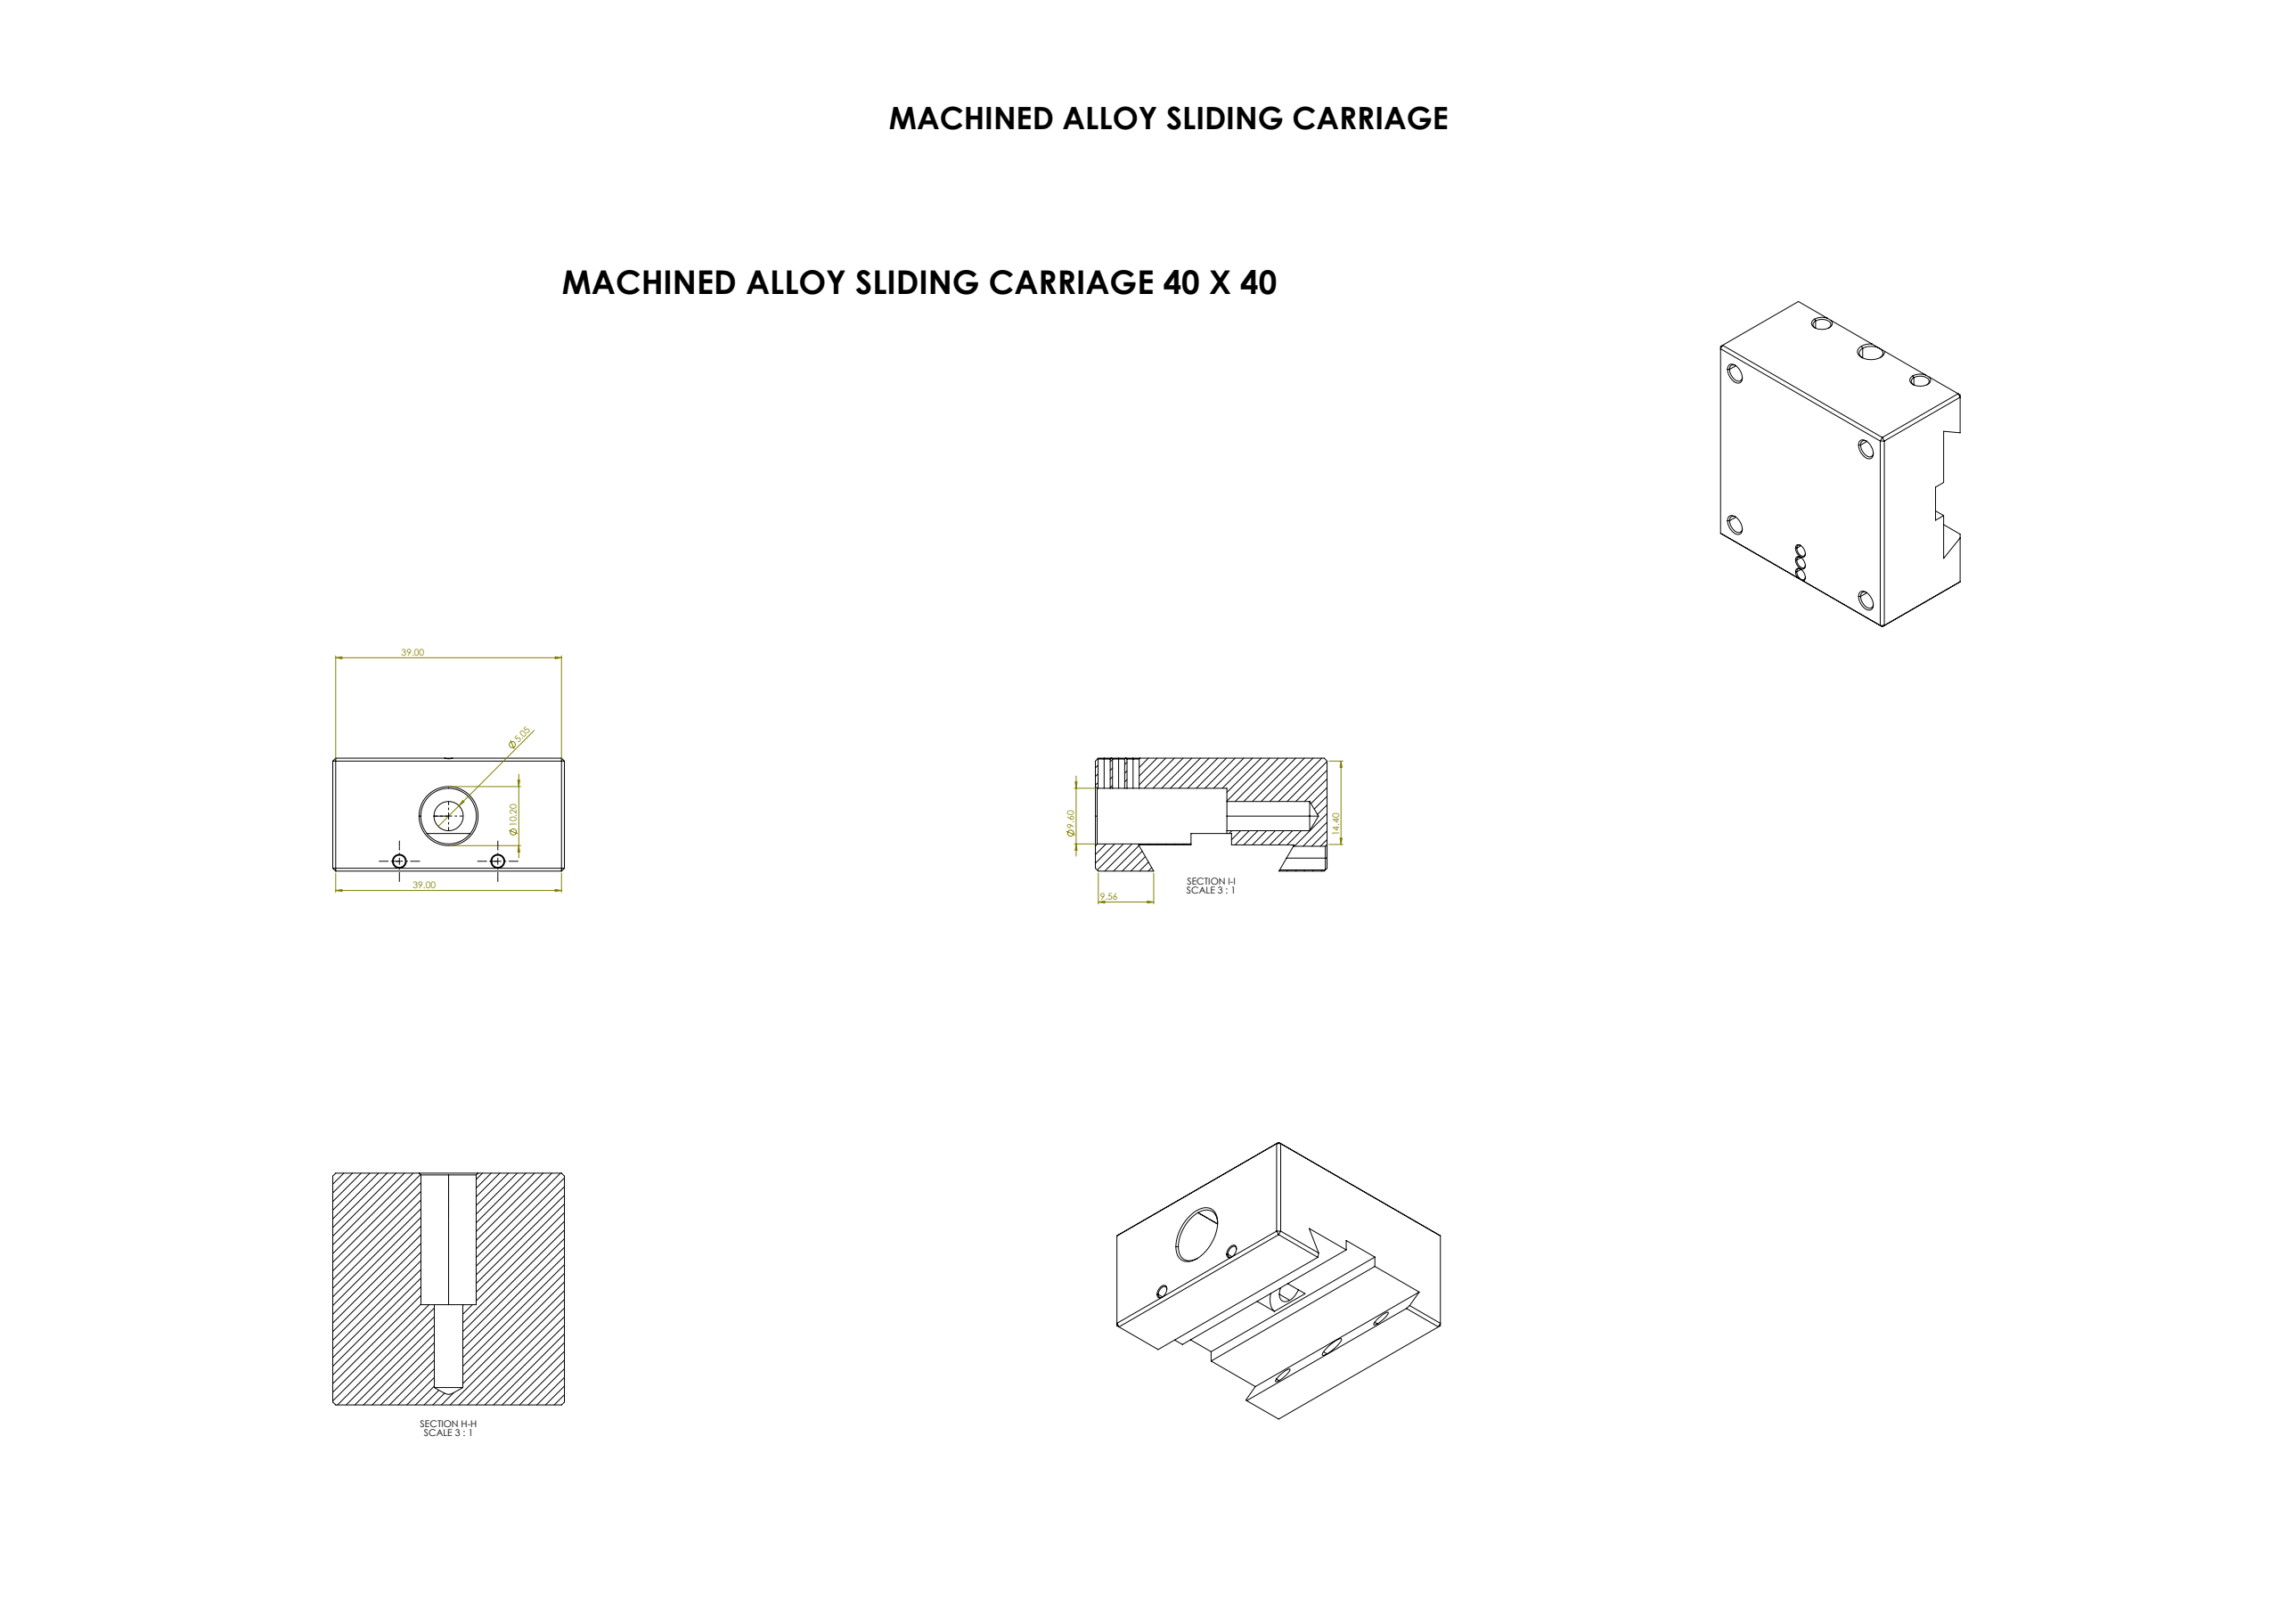
ISO-10303-21;
HEADER;
/* Generated by software containing ST-Developer
 * from STEP Tools, Inc. (www.steptools.com) 
 */

FILE_DESCRIPTION(
/* description */ (''),
/* implementation_level */ '2;1');

FILE_NAME(
/* name */ 'Machined Alloy Sliding Carriage 40 x 40.step',
/* time_stamp */ '2026-10-05T09:57:53+05:00',
/* author */ (''),
/* organization */ (''),
/* preprocessor_version */ 'ST-DEVELOPER v20.2',
/* originating_system */ 'Autodesk Translation Framework v15.15.0.0',
/* authorisation */ '');

FILE_SCHEMA (('AUTOMOTIVE_DESIGN { 1 0 10303 214 3 1 1 }'));
ENDSEC;

DATA;
#10=MECHANICAL_DESIGN_GEOMETRIC_PRESENTATION_REPRESENTATION('',(#552),#113984);
#142=(
BOUNDED_CURVE()
B_SPLINE_CURVE(2,(#92151,#92152,#92153),.UNSPECIFIED.,.F.,.F.)
B_SPLINE_CURVE_WITH_KNOTS((3,3),(0.,0.16248076809272),.UNSPECIFIED.)
CURVE()
GEOMETRIC_REPRESENTATION_ITEM()
RATIONAL_B_SPLINE_CURVE((1.,1.,1.))
REPRESENTATION_ITEM('')
);
#143=(
BOUNDED_CURVE()
B_SPLINE_CURVE(2,(#92201,#92202,#92203),.UNSPECIFIED.,.F.,.F.)
B_SPLINE_CURVE_WITH_KNOTS((3,3),(0.,0.0845576726264383),.UNSPECIFIED.)
CURVE()
GEOMETRIC_REPRESENTATION_ITEM()
RATIONAL_B_SPLINE_CURVE((1.,1.,1.))
REPRESENTATION_ITEM('')
);
#144=(
BOUNDED_CURVE()
B_SPLINE_CURVE(2,(#92222,#92223,#92224),.UNSPECIFIED.,.F.,.F.)
B_SPLINE_CURVE_WITH_KNOTS((3,3),(0.,0.0845576726264383),.UNSPECIFIED.)
CURVE()
GEOMETRIC_REPRESENTATION_ITEM()
RATIONAL_B_SPLINE_CURVE((1.,1.,1.))
REPRESENTATION_ITEM('')
);
#145=(
BOUNDED_CURVE()
B_SPLINE_CURVE(2,(#92227,#92228,#92229),.UNSPECIFIED.,.F.,.F.)
B_SPLINE_CURVE_WITH_KNOTS((3,3),(0.16248076809272,0.324961536185439),
 .UNSPECIFIED.)
CURVE()
GEOMETRIC_REPRESENTATION_ITEM()
RATIONAL_B_SPLINE_CURVE((1.,1.,1.))
REPRESENTATION_ITEM('')
);
#146=(
BOUNDED_CURVE()
B_SPLINE_CURVE(2,(#92262,#92263,#92264),.UNSPECIFIED.,.F.,.F.)
B_SPLINE_CURVE_WITH_KNOTS((3,3),(0.,0.13564659966251),.UNSPECIFIED.)
CURVE()
GEOMETRIC_REPRESENTATION_ITEM()
RATIONAL_B_SPLINE_CURVE((1.,1.,1.))
REPRESENTATION_ITEM('')
);
#516=SHAPE_REPRESENTATION_RELATIONSHIP('SRR','None',#114053,#534);
#534=ADVANCED_BREP_SHAPE_REPRESENTATION('',(#570),#113967);
#552=STYLED_ITEM('',(#114324),#570);
#570=MANIFOLD_SOLID_BREP('Machined Alloy Sliding Carriage 40 x 40',#60393);
#595=ELLIPSE('',#61838,1.78978583448783,1.54999999999999);
#596=ELLIPSE('',#61844,1.78978583448783,1.54999999999999);
#597=ELLIPSE('',#61849,2.36713610367747,2.05);
#621=CYLINDRICAL_SURFACE('',#61824,1.05);
#622=CYLINDRICAL_SURFACE('',#61828,1.05);
#623=CYLINDRICAL_SURFACE('',#61837,1.54999999999999);
#624=CYLINDRICAL_SURFACE('',#61843,1.54999999999999);
#625=CYLINDRICAL_SURFACE('',#61848,2.05);
#626=CYLINDRICAL_SURFACE('',#61856,1.05);
#627=CYLINDRICAL_SURFACE('',#61869,1.05);
#628=CYLINDRICAL_SURFACE('',#61875,1.05);
#629=CYLINDRICAL_SURFACE('',#61887,1.54999999999999);
#630=CYLINDRICAL_SURFACE('',#61891,1.54999999999999);
#631=CYLINDRICAL_SURFACE('',#61895,1.54999999999999);
#632=CYLINDRICAL_SURFACE('',#61899,1.54999999999999);
#633=CYLINDRICAL_SURFACE('',#61908,4.8);
#634=CYLINDRICAL_SURFACE('',#61914,2.525);
#887=CONICAL_SURFACE('',#61813,2.2,0.785398163397448);
#888=CONICAL_SURFACE('',#61816,1.12500000000001,0.785398163397478);
#889=CONICAL_SURFACE('',#61826,1.12500000000001,0.785398163397478);
#890=CONICAL_SURFACE('',#61830,0.525000000000002,1.02974425867666);
#891=CONICAL_SURFACE('',#61831,0.525000000000002,1.02974425867665);
#892=CONICAL_SURFACE('',#61832,1.675,0.785398163397455);
#893=CONICAL_SURFACE('',#61839,1.675,0.785398163397455);
#894=CONICAL_SURFACE('',#61845,2.2,0.785398163397448);
#895=CONICAL_SURFACE('',#61851,1.125,0.785398163397434);
#896=CONICAL_SURFACE('',#61860,1.12500000000001,0.785398163397463);
#897=CONICAL_SURFACE('',#61873,1.12500000000001,0.785398163397463);
#898=CONICAL_SURFACE('',#61885,1.675,0.785398163397457);
#899=CONICAL_SURFACE('',#61889,1.675,0.785398163397457);
#900=CONICAL_SURFACE('',#61893,1.675,0.785398163397457);
#901=CONICAL_SURFACE('',#61897,1.675,0.785398163397457);
#902=CONICAL_SURFACE('',#61901,1.54999999999999,1.02974425867665);
#903=CONICAL_SURFACE('',#61902,1.54999999999999,1.02974425867665);
#904=CONICAL_SURFACE('',#61903,1.54999999999999,1.02974425867665);
#905=CONICAL_SURFACE('',#61904,1.54999999999999,1.02974425867665);
#906=CONICAL_SURFACE('',#61905,4.95,0.785398163397434);
#907=CONICAL_SURFACE('',#61912,1.26250000000001,1.02974425867666);
#1001=CIRCLE('',#61814,2.35);
#1002=CIRCLE('',#61815,2.05);
#1003=CIRCLE('',#61817,1.20000000000001);
#1004=CIRCLE('',#61818,1.05);
#1005=CIRCLE('',#61819,1.20000000000001);
#1006=CIRCLE('',#61821,1.20000000000001);
#1007=CIRCLE('',#61822,1.20000000000001);
#1008=CIRCLE('',#61823,5.1);
#1009=CIRCLE('',#61825,1.05);
#1010=CIRCLE('',#61827,1.05);
#1011=CIRCLE('',#61829,1.05);
#1012=CIRCLE('',#61833,1.8);
#1013=CIRCLE('',#61834,1.54999999999999);
#1014=CIRCLE('',#61835,1.8);
#1015=CIRCLE('',#61840,1.8);
#1016=CIRCLE('',#61841,1.54999999999999);
#1017=CIRCLE('',#61842,1.8);
#1018=CIRCLE('',#61846,2.05);
#1019=CIRCLE('',#61847,2.35);
#1020=CIRCLE('',#61852,1.2);
#1021=CIRCLE('',#61853,1.05);
#1022=CIRCLE('',#61854,1.2);
#1023=CIRCLE('',#61857,1.05);
#1024=CIRCLE('',#61858,1.05);
#1025=CIRCLE('',#61859,1.05);
#1026=CIRCLE('',#61861,1.20000000000001);
#1027=CIRCLE('',#61862,1.05);
#1028=CIRCLE('',#61864,1.20000000000001);
#1029=CIRCLE('',#61865,1.8);
#1030=CIRCLE('',#61866,1.8);
#1031=CIRCLE('',#61867,1.8);
#1032=CIRCLE('',#61868,1.8);
#1033=CIRCLE('',#61870,1.05);
#1034=CIRCLE('',#61871,1.05);
#1035=CIRCLE('',#61872,1.05);
#1036=CIRCLE('',#61874,1.05);
#1037=CIRCLE('',#61876,1.05);
#1038=CIRCLE('',#61877,1.05);
#1039=CIRCLE('',#61878,1.05);
#1040=CIRCLE('',#61886,1.54999999999999);
#1041=CIRCLE('',#61888,1.54999999999999);
#1042=CIRCLE('',#61890,1.54999999999999);
#1043=CIRCLE('',#61892,1.54999999999999);
#1044=CIRCLE('',#61894,1.54999999999999);
#1045=CIRCLE('',#61896,1.54999999999999);
#1046=CIRCLE('',#61898,1.54999999999999);
#1047=CIRCLE('',#61900,1.54999999999999);
#1048=CIRCLE('',#61906,4.8);
#1049=CIRCLE('',#61907,4.8);
#1050=CIRCLE('',#61909,4.8);
#1051=CIRCLE('',#61910,4.8);
#1052=CIRCLE('',#61911,4.8);
#1053=CIRCLE('',#61913,2.525);
#1054=CIRCLE('',#61915,2.525);
#1811=FACE_BOUND('',#9411,.T.);
#1812=FACE_BOUND('',#9430,.T.);
#1813=FACE_BOUND('',#9431,.T.);
#1814=FACE_BOUND('',#9432,.T.);
#1815=FACE_BOUND('',#9433,.T.);
#1816=FACE_BOUND('',#9434,.T.);
#1817=FACE_BOUND('',#9435,.T.);
#1818=FACE_BOUND('',#9462,.T.);
#1819=FACE_BOUND('',#9470,.T.);
#1820=FACE_BOUND('',#9471,.T.);
#1821=FACE_BOUND('',#9472,.T.);
#2978=PLANE('',#61820);
#2979=PLANE('',#61836);
#2980=PLANE('',#61850);
#2981=PLANE('',#61855);
#2982=PLANE('',#61863);
#2983=PLANE('',#61879);
#2984=PLANE('',#61880);
#2985=PLANE('',#61881);
#2986=PLANE('',#61882);
#2987=PLANE('',#61883);
#2988=PLANE('',#61884);
#2989=PLANE('',#61916);
#2990=PLANE('',#61917);
#2991=PLANE('',#61918);
#2992=PLANE('',#61919);
#2993=PLANE('',#61920);
#2994=PLANE('',#61921);
#2995=PLANE('',#61922);
#2996=PLANE('',#61923);
#2997=PLANE('',#61924);
#2998=PLANE('',#61925);
#2999=PLANE('',#61926);
#3000=PLANE('',#61927);
#3001=PLANE('',#61928);
#3002=PLANE('',#61929);
#3003=PLANE('',#61930);
#3004=PLANE('',#61931);
#3005=PLANE('',#61932);
#3006=PLANE('',#61933);
#3007=PLANE('',#61934);
#3008=PLANE('',#61935);
#3009=PLANE('',#61936);
#3010=PLANE('',#61937);
#3011=PLANE('',#61938);
#3012=PLANE('',#61939);
#3013=PLANE('',#61940);
#3014=PLANE('',#61941);
#3015=PLANE('',#61942);
#3016=PLANE('',#61943);
#3017=PLANE('',#61944);
#3018=PLANE('',#61945);
#3019=PLANE('',#61946);
#3020=PLANE('',#61947);
#5872=FACE_OUTER_BOUND('',#9408,.T.);
#5873=FACE_OUTER_BOUND('',#9409,.T.);
#5874=FACE_OUTER_BOUND('',#9410,.T.);
#5875=FACE_OUTER_BOUND('',#9412,.T.);
#5876=FACE_OUTER_BOUND('',#9413,.T.);
#5877=FACE_OUTER_BOUND('',#9414,.T.);
#5878=FACE_OUTER_BOUND('',#9415,.T.);
#5879=FACE_OUTER_BOUND('',#9416,.T.);
#5880=FACE_OUTER_BOUND('',#9417,.T.);
#5881=FACE_OUTER_BOUND('',#9418,.T.);
#5882=FACE_OUTER_BOUND('',#9419,.T.);
#5883=FACE_OUTER_BOUND('',#9420,.T.);
#5884=FACE_OUTER_BOUND('',#9421,.T.);
#5885=FACE_OUTER_BOUND('',#9422,.T.);
#5886=FACE_OUTER_BOUND('',#9423,.T.);
#5887=FACE_OUTER_BOUND('',#9424,.T.);
#5888=FACE_OUTER_BOUND('',#9425,.T.);
#5889=FACE_OUTER_BOUND('',#9426,.T.);
#5890=FACE_OUTER_BOUND('',#9427,.T.);
#5891=FACE_OUTER_BOUND('',#9428,.T.);
#5892=FACE_OUTER_BOUND('',#9429,.T.);
#5893=FACE_OUTER_BOUND('',#9436,.T.);
#5894=FACE_OUTER_BOUND('',#9437,.T.);
#5895=FACE_OUTER_BOUND('',#9438,.T.);
#5896=FACE_OUTER_BOUND('',#9439,.T.);
#5897=FACE_OUTER_BOUND('',#9440,.T.);
#5898=FACE_OUTER_BOUND('',#9441,.T.);
#5899=FACE_OUTER_BOUND('',#9442,.T.);
#5900=FACE_OUTER_BOUND('',#9443,.T.);
#5901=FACE_OUTER_BOUND('',#9444,.T.);
#5902=FACE_OUTER_BOUND('',#9445,.T.);
#5903=FACE_OUTER_BOUND('',#9446,.T.);
#5904=FACE_OUTER_BOUND('',#9447,.T.);
#5905=FACE_OUTER_BOUND('',#9448,.T.);
#5906=FACE_OUTER_BOUND('',#9449,.T.);
#5907=FACE_OUTER_BOUND('',#9450,.T.);
#5908=FACE_OUTER_BOUND('',#9451,.T.);
#5909=FACE_OUTER_BOUND('',#9452,.T.);
#5910=FACE_OUTER_BOUND('',#9453,.T.);
#5911=FACE_OUTER_BOUND('',#9454,.T.);
#5912=FACE_OUTER_BOUND('',#9455,.T.);
#5913=FACE_OUTER_BOUND('',#9456,.T.);
#5914=FACE_OUTER_BOUND('',#9457,.T.);
#5915=FACE_OUTER_BOUND('',#9458,.T.);
#5916=FACE_OUTER_BOUND('',#9459,.T.);
#5917=FACE_OUTER_BOUND('',#9460,.T.);
#5918=FACE_OUTER_BOUND('',#9461,.T.);
#5919=FACE_OUTER_BOUND('',#9463,.T.);
#5920=FACE_OUTER_BOUND('',#9464,.T.);
#5921=FACE_OUTER_BOUND('',#9465,.T.);
#5922=FACE_OUTER_BOUND('',#9466,.T.);
#5923=FACE_OUTER_BOUND('',#9467,.T.);
#5924=FACE_OUTER_BOUND('',#9468,.T.);
#5925=FACE_OUTER_BOUND('',#9469,.T.);
#5926=FACE_OUTER_BOUND('',#9473,.T.);
#5927=FACE_OUTER_BOUND('',#9474,.T.);
#5928=FACE_OUTER_BOUND('',#9475,.T.);
#5929=FACE_OUTER_BOUND('',#9476,.T.);
#5930=FACE_OUTER_BOUND('',#9477,.T.);
#5931=FACE_OUTER_BOUND('',#9478,.T.);
#5932=FACE_OUTER_BOUND('',#9479,.T.);
#5933=FACE_OUTER_BOUND('',#9480,.T.);
#5934=FACE_OUTER_BOUND('',#9481,.T.);
#5935=FACE_OUTER_BOUND('',#9482,.T.);
#5936=FACE_OUTER_BOUND('',#9483,.T.);
#5937=FACE_OUTER_BOUND('',#9484,.T.);
#5938=FACE_OUTER_BOUND('',#9485,.T.);
#5939=FACE_OUTER_BOUND('',#9486,.T.);
#5940=FACE_OUTER_BOUND('',#9487,.T.);
#5941=FACE_OUTER_BOUND('',#9488,.T.);
#5942=FACE_OUTER_BOUND('',#9489,.T.);
#5943=FACE_OUTER_BOUND('',#9490,.T.);
#5944=FACE_OUTER_BOUND('',#9491,.T.);
#5945=FACE_OUTER_BOUND('',#9492,.T.);
#5946=FACE_OUTER_BOUND('',#9493,.T.);
#5947=FACE_OUTER_BOUND('',#9494,.T.);
#5948=FACE_OUTER_BOUND('',#9495,.T.);
#5949=FACE_OUTER_BOUND('',#9496,.T.);
#9408=EDGE_LOOP('',(#48495,#48496,#48497,#48498));
#9409=EDGE_LOOP('',(#48499,#48500,#48501,#48502,#48503));
#9410=EDGE_LOOP('',(#48504,#48505,#48506,#48507,#48508,#48509,#48510,#48511,
#48512,#48513));
#9411=EDGE_LOOP('',(#48514));
#9412=EDGE_LOOP('',(#48515,#48516,#48517,#48518));
#9413=EDGE_LOOP('',(#48519,#48520,#48521,#48522,#48523));
#9414=EDGE_LOOP('',(#48524,#48525,#48526,#48527));
#9415=EDGE_LOOP('',(#48528,#48529,#48530));
#9416=EDGE_LOOP('',(#48531,#48532,#48533));
#9417=EDGE_LOOP('',(#48534,#48535,#48536,#48537,#48538,#48539));
#9418=EDGE_LOOP('',(#48540,#48541,#48542,#48543,#48544,#48545,#48546,#48547,
#48548,#48549,#48550));
#9419=EDGE_LOOP('',(#48551,#48552,#48553,#48554));
#9420=EDGE_LOOP('',(#48555,#48556,#48557,#48558,#48559,#48560));
#9421=EDGE_LOOP('',(#48561,#48562,#48563,#48564));
#9422=EDGE_LOOP('',(#48565,#48566,#48567,#48568));
#9423=EDGE_LOOP('',(#48569,#48570,#48571,#48572,#48573));
#9424=EDGE_LOOP('',(#48574,#48575,#48576,#48577,#48578,#48579,#48580,#48581,
#48582,#48583,#48584,#48585,#48586));
#9425=EDGE_LOOP('',(#48587,#48588,#48589,#48590,#48591,#48592));
#9426=EDGE_LOOP('',(#48593,#48594,#48595,#48596,#48597,#48598));
#9427=EDGE_LOOP('',(#48599,#48600,#48601,#48602,#48603,#48604));
#9428=EDGE_LOOP('',(#48605,#48606,#48607,#48608));
#9429=EDGE_LOOP('',(#48609,#48610,#48611,#48612,#48613,#48614,#48615));
#9430=EDGE_LOOP('',(#48616));
#9431=EDGE_LOOP('',(#48617));
#9432=EDGE_LOOP('',(#48618));
#9433=EDGE_LOOP('',(#48619));
#9434=EDGE_LOOP('',(#48620));
#9435=EDGE_LOOP('',(#48621));
#9436=EDGE_LOOP('',(#48622,#48623,#48624,#48625,#48626,#48627));
#9437=EDGE_LOOP('',(#48628,#48629,#48630,#48631));
#9438=EDGE_LOOP('',(#48632,#48633,#48634,#48635,#48636,#48637));
#9439=EDGE_LOOP('',(#48638,#48639));
#9440=EDGE_LOOP('',(#48640,#48641,#48642));
#9441=EDGE_LOOP('',(#48643,#48644));
#9442=EDGE_LOOP('',(#48645,#48646,#48647));
#9443=EDGE_LOOP('',(#48648,#48649));
#9444=EDGE_LOOP('',(#48650,#48651,#48652));
#9445=EDGE_LOOP('',(#48653,#48654,#48655,#48656));
#9446=EDGE_LOOP('',(#48657,#48658,#48659,#48660));
#9447=EDGE_LOOP('',(#48661,#48662,#48663,#48664));
#9448=EDGE_LOOP('',(#48665,#48666,#48667,#48668));
#9449=EDGE_LOOP('',(#48669,#48670,#48671,#48672));
#9450=EDGE_LOOP('',(#48673,#48674,#48675,#48676));
#9451=EDGE_LOOP('',(#48677,#48678,#48679,#48680));
#9452=EDGE_LOOP('',(#48681,#48682,#48683,#48684));
#9453=EDGE_LOOP('',(#48685,#48686,#48687));
#9454=EDGE_LOOP('',(#48688,#48689,#48690));
#9455=EDGE_LOOP('',(#48691,#48692,#48693));
#9456=EDGE_LOOP('',(#48694,#48695,#48696));
#9457=EDGE_LOOP('',(#48697,#48698,#48699,#48700,#48701));
#9458=EDGE_LOOP('',(#48702,#48703,#48704,#48705,#48706,#48707,#48708,#48709,
#48710,#48711,#48712,#48713,#48714,#48715,#48716,#48717,#48718,#48719,#48720,
#48721,#48722));
#9459=EDGE_LOOP('',(#48723,#48724,#48725));
#9460=EDGE_LOOP('',(#48726,#48727,#48728,#48729));
#9461=EDGE_LOOP('',(#48730,#48731,#48732));
#9462=EDGE_LOOP('',(#48733));
#9463=EDGE_LOOP('',(#48734,#48735,#48736,#48737,#48738,#48739,#48740,#48741));
#9464=EDGE_LOOP('',(#48742,#48743,#48744,#48745));
#9465=EDGE_LOOP('',(#48746,#48747,#48748,#48749,#48750,#48751));
#9466=EDGE_LOOP('',(#48752,#48753,#48754,#48755,#48756,#48757,#48758,#48759,
#48760,#48761,#48762,#48763));
#9467=EDGE_LOOP('',(#48764,#48765,#48766,#48767));
#9468=EDGE_LOOP('',(#48768,#48769,#48770,#48771,#48772,#48773));
#9469=EDGE_LOOP('',(#48774,#48775,#48776,#48777,#48778,#48779));
#9470=EDGE_LOOP('',(#48780));
#9471=EDGE_LOOP('',(#48781));
#9472=EDGE_LOOP('',(#48782));
#9473=EDGE_LOOP('',(#48783,#48784,#48785,#48786));
#9474=EDGE_LOOP('',(#48787,#48788,#48789,#48790));
#9475=EDGE_LOOP('',(#48791,#48792,#48793,#48794));
#9476=EDGE_LOOP('',(#48795,#48796,#48797,#48798));
#9477=EDGE_LOOP('',(#48799,#48800,#48801,#48802));
#9478=EDGE_LOOP('',(#48803,#48804,#48805));
#9479=EDGE_LOOP('',(#48806,#48807,#48808));
#9480=EDGE_LOOP('',(#48809,#48810,#48811));
#9481=EDGE_LOOP('',(#48812,#48813,#48814));
#9482=EDGE_LOOP('',(#48815,#48816,#48817));
#9483=EDGE_LOOP('',(#48818,#48819,#48820));
#9484=EDGE_LOOP('',(#48821,#48822,#48823));
#9485=EDGE_LOOP('',(#48824,#48825,#48826));
#9486=EDGE_LOOP('',(#48827,#48828,#48829,#48830));
#9487=EDGE_LOOP('',(#48831,#48832,#48833,#48834));
#9488=EDGE_LOOP('',(#48835,#48836,#48837,#48838));
#9489=EDGE_LOOP('',(#48839,#48840,#48841,#48842));
#9490=EDGE_LOOP('',(#48843,#48844,#48845,#48846));
#9491=EDGE_LOOP('',(#48847,#48848,#48849,#48850));
#9492=EDGE_LOOP('',(#48851,#48852,#48853,#48854));
#9493=EDGE_LOOP('',(#48855,#48856,#48857,#48858,#48859,#48860));
#9494=EDGE_LOOP('',(#48861,#48862,#48863,#48864));
#9495=EDGE_LOOP('',(#48865,#48866,#48867,#48868));
#9496=EDGE_LOOP('',(#48869,#48870,#48871,#48872,#48873,#48874,#48875,#48876,
#48877,#48878,#48879,#48880));
#14156=LINE('',#92147,#20190);
#14157=LINE('',#92160,#20191);
#14158=LINE('',#92166,#20192);
#14159=LINE('',#92168,#20193);
#14160=LINE('',#92172,#20194);
#14161=LINE('',#92174,#20195);
#14162=LINE('',#92176,#20196);
#14163=LINE('',#92177,#20197);
#14164=LINE('',#92182,#20198);
#14165=LINE('',#92186,#20199);
#14166=LINE('',#92190,#20200);
#14167=LINE('',#92194,#20201);
#14168=LINE('',#92197,#20202);
#14169=LINE('',#92207,#20203);
#14170=LINE('',#92212,#20204);
#14171=LINE('',#92214,#20205);
#14172=LINE('',#92216,#20206);
#14173=LINE('',#92218,#20207);
#14174=LINE('',#92220,#20208);
#14175=LINE('',#92226,#20209);
#14176=LINE('',#92230,#20210);
#14177=LINE('',#92233,#20211);
#14178=LINE('',#92239,#20212);
#14179=LINE('',#92244,#20213);
#14180=LINE('',#92251,#20214);
#14181=LINE('',#92255,#20215);
#14182=LINE('',#92257,#20216);
#14183=LINE('',#92258,#20217);
#14184=LINE('',#92268,#20218);
#14185=LINE('',#92273,#20219);
#14186=LINE('',#92274,#20220);
#14187=LINE('',#92276,#20221);
#14188=LINE('',#92277,#20222);
#14189=LINE('',#92280,#20223);
#14190=LINE('',#92290,#20224);
#14191=LINE('',#92294,#20225);
#14192=LINE('',#92296,#20226);
#14193=LINE('',#92297,#20227);
#14194=LINE('',#92310,#20228);
#14195=LINE('',#92318,#20229);
#14196=LINE('',#92322,#20230);
#14197=LINE('',#92329,#20231);
#14198=LINE('',#92331,#20232);
#14199=LINE('',#92333,#20233);
#14200=LINE('',#92335,#20234);
#14201=LINE('',#92337,#20235);
#14202=LINE('',#92339,#20236);
#14203=LINE('',#92342,#20237);
#14204=LINE('',#92346,#20238);
#14205=LINE('',#92350,#20239);
#14206=LINE('',#92354,#20240);
#14207=LINE('',#92358,#20241);
#14208=LINE('',#92362,#20242);
#14209=LINE('',#92366,#20243);
#14210=LINE('',#92370,#20244);
#14211=LINE('',#92374,#20245);
#14212=LINE('',#92377,#20246);
#14213=LINE('',#92380,#20247);
#14214=LINE('',#92383,#20248);
#14215=LINE('',#92386,#20249);
#14216=LINE('',#92391,#20250);
#14217=LINE('',#92392,#20251);
#14218=LINE('',#92393,#20252);
#14219=LINE('',#92395,#20253);
#14220=LINE('',#92399,#20254);
#14221=LINE('',#92403,#20255);
#14222=LINE('',#92408,#20256);
#14223=LINE('',#92413,#20257);
#14224=LINE('',#92415,#20258);
#14225=LINE('',#92418,#20259);
#14226=LINE('',#92420,#20260);
#14227=LINE('',#92422,#20261);
#14228=LINE('',#92424,#20262);
#14229=LINE('',#92425,#20263);
#14230=LINE('',#92429,#20264);
#14231=LINE('',#92430,#20265);
#14232=LINE('',#92431,#20266);
#14233=LINE('',#92434,#20267);
#14234=LINE('',#92436,#20268);
#14235=LINE('',#92437,#20269);
#14236=LINE('',#92440,#20270);
#14237=LINE('',#92442,#20271);
#14238=LINE('',#92444,#20272);
#14239=LINE('',#92446,#20273);
#14240=LINE('',#92448,#20274);
#14241=LINE('',#92450,#20275);
#14242=LINE('',#92452,#20276);
#14243=LINE('',#92454,#20277);
#14244=LINE('',#92455,#20278);
#14245=LINE('',#92458,#20279);
#14246=LINE('',#92459,#20280);
#14247=LINE('',#92462,#20281);
#14248=LINE('',#92464,#20282);
#14249=LINE('',#92466,#20283);
#14250=LINE('',#92467,#20284);
#14251=LINE('',#92470,#20285);
#14252=LINE('',#92472,#20286);
#14253=LINE('',#92474,#20287);
#14254=LINE('',#92476,#20288);
#14255=LINE('',#92477,#20289);
#14256=LINE('',#92479,#20290);
#14257=LINE('',#92482,#20291);
#14258=LINE('',#92483,#20292);
#14259=LINE('',#92485,#20293);
#14260=LINE('',#92486,#20294);
#14261=LINE('',#92489,#20295);
#14262=LINE('',#92490,#20296);
#14263=LINE('',#92493,#20297);
#14264=LINE('',#92494,#20298);
#14265=LINE('',#92496,#20299);
#14266=LINE('',#92497,#20300);
#14267=LINE('',#92500,#20301);
#14268=LINE('',#92501,#20302);
#14269=LINE('',#92503,#20303);
#14270=LINE('',#92504,#20304);
#14271=LINE('',#92507,#20305);
#14272=LINE('',#92508,#20306);
#14273=LINE('',#92510,#20307);
#14274=LINE('',#92511,#20308);
#14275=LINE('',#92514,#20309);
#14276=LINE('',#92515,#20310);
#14277=LINE('',#92516,#20311);
#14278=LINE('',#92518,#20312);
#14279=LINE('',#92520,#20313);
#14280=LINE('',#92521,#20314);
#14281=LINE('',#92522,#20315);
#14282=LINE('',#92527,#20316);
#14283=LINE('',#92529,#20317);
#14284=LINE('',#92532,#20318);
#14285=LINE('',#92533,#20319);
#14286=LINE('',#92536,#20320);
#20190=VECTOR('',#69466,2.2);
#20191=VECTOR('',#69475,1.12500000000001);
#20192=VECTOR('',#69482,10.);
#20193=VECTOR('',#69483,10.);
#20194=VECTOR('',#69488,10.);
#20195=VECTOR('',#69489,10.);
#20196=VECTOR('',#69490,10.);
#20197=VECTOR('',#69491,10.);
#20198=VECTOR('',#69496,1.05);
#20199=VECTOR('',#69501,1.12500000000001);
#20200=VECTOR('',#69506,1.05);
#20201=VECTOR('',#69511,0.525000000000002);
#20202=VECTOR('',#69514,0.525000000000002);
#20203=VECTOR('',#69519,1.675);
#20204=VECTOR('',#69526,10.);
#20205=VECTOR('',#69527,10.);
#20206=VECTOR('',#69528,10.);
#20207=VECTOR('',#69529,10.);
#20208=VECTOR('',#69530,10.);
#20209=VECTOR('',#69531,10.);
#20210=VECTOR('',#69532,10.);
#20211=VECTOR('',#69535,1.54999999999999);
#20212=VECTOR('',#69542,1.675);
#20213=VECTOR('',#69549,1.54999999999999);
#20214=VECTOR('',#69560,2.05);
#20215=VECTOR('',#69565,10.);
#20216=VECTOR('',#69566,10.);
#20217=VECTOR('',#69567,10.);
#20218=VECTOR('',#69572,1.125);
#20219=VECTOR('',#69579,10.);
#20220=VECTOR('',#69580,10.);
#20221=VECTOR('',#69581,10.);
#20222=VECTOR('',#69582,10.);
#20223=VECTOR('',#69585,1.05);
#20224=VECTOR('',#69596,1.12500000000001);
#20225=VECTOR('',#69601,10.);
#20226=VECTOR('',#69602,10.);
#20227=VECTOR('',#69603,10.);
#20228=VECTOR('',#69616,1.05);
#20229=VECTOR('',#69625,1.12500000000001);
#20230=VECTOR('',#69630,1.05);
#20231=VECTOR('',#69639,10.);
#20232=VECTOR('',#69642,10.);
#20233=VECTOR('',#69645,10.);
#20234=VECTOR('',#69648,10.);
#20235=VECTOR('',#69651,10.);
#20236=VECTOR('',#69654,10.);
#20237=VECTOR('',#69657,1.675);
#20238=VECTOR('',#69662,1.54999999999999);
#20239=VECTOR('',#69667,1.675);
#20240=VECTOR('',#69672,1.54999999999999);
#20241=VECTOR('',#69677,1.675);
#20242=VECTOR('',#69682,1.54999999999999);
#20243=VECTOR('',#69687,1.675);
#20244=VECTOR('',#69692,1.54999999999999);
#20245=VECTOR('',#69697,1.54999999999999);
#20246=VECTOR('',#69700,1.54999999999999);
#20247=VECTOR('',#69703,1.54999999999999);
#20248=VECTOR('',#69706,1.54999999999999);
#20249=VECTOR('',#69709,4.95);
#20250=VECTOR('',#69716,4.8);
#20251=VECTOR('',#69717,4.8);
#20252=VECTOR('',#69718,4.8);
#20253=VECTOR('',#69719,4.8);
#20254=VECTOR('',#69722,10.);
#20255=VECTOR('',#69725,10.);
#20256=VECTOR('',#69730,1.26250000000001);
#20257=VECTOR('',#69737,2.525);
#20258=VECTOR('',#69740,10.);
#20259=VECTOR('',#69743,10.);
#20260=VECTOR('',#69744,10.);
#20261=VECTOR('',#69745,10.);
#20262=VECTOR('',#69746,10.);
#20263=VECTOR('',#69747,10.);
#20264=VECTOR('',#69750,10.);
#20265=VECTOR('',#69751,10.);
#20266=VECTOR('',#69752,10.);
#20267=VECTOR('',#69755,10.);
#20268=VECTOR('',#69756,10.);
#20269=VECTOR('',#69757,10.);
#20270=VECTOR('',#69760,10.);
#20271=VECTOR('',#69761,10.);
#20272=VECTOR('',#69762,10.);
#20273=VECTOR('',#69763,10.);
#20274=VECTOR('',#69764,10.);
#20275=VECTOR('',#69765,10.);
#20276=VECTOR('',#69766,10.);
#20277=VECTOR('',#69767,10.);
#20278=VECTOR('',#69768,10.);
#20279=VECTOR('',#69771,10.);
#20280=VECTOR('',#69772,10.);
#20281=VECTOR('',#69775,10.);
#20282=VECTOR('',#69776,10.);
#20283=VECTOR('',#69777,10.);
#20284=VECTOR('',#69778,10.);
#20285=VECTOR('',#69781,10.);
#20286=VECTOR('',#69782,10.);
#20287=VECTOR('',#69783,10.);
#20288=VECTOR('',#69784,10.);
#20289=VECTOR('',#69785,10.);
#20290=VECTOR('',#69788,10.);
#20291=VECTOR('',#69791,10.);
#20292=VECTOR('',#69792,10.);
#20293=VECTOR('',#69795,10.);
#20294=VECTOR('',#69796,10.);
#20295=VECTOR('',#69799,10.);
#20296=VECTOR('',#69800,10.);
#20297=VECTOR('',#69803,10.);
#20298=VECTOR('',#69804,10.);
#20299=VECTOR('',#69807,10.);
#20300=VECTOR('',#69808,10.);
#20301=VECTOR('',#69811,10.);
#20302=VECTOR('',#69812,10.);
#20303=VECTOR('',#69815,10.);
#20304=VECTOR('',#69816,10.);
#20305=VECTOR('',#69819,10.);
#20306=VECTOR('',#69820,10.);
#20307=VECTOR('',#69823,10.);
#20308=VECTOR('',#69824,10.);
#20309=VECTOR('',#69827,10.);
#20310=VECTOR('',#69828,10.);
#20311=VECTOR('',#69829,10.);
#20312=VECTOR('',#69832,10.);
#20313=VECTOR('',#69835,10.);
#20314=VECTOR('',#69836,10.);
#20315=VECTOR('',#69837,10.);
#20316=VECTOR('',#69846,10.);
#20317=VECTOR('',#69849,10.);
#20318=VECTOR('',#69854,10.);
#20319=VECTOR('',#69855,10.);
#20320=VECTOR('',#69860,10.);
#27763=VERTEX_POINT('',#92145);
#27764=VERTEX_POINT('',#92146);
#27765=VERTEX_POINT('',#92148);
#27766=VERTEX_POINT('',#92150);
#27767=VERTEX_POINT('',#92156);
#27768=VERTEX_POINT('',#92157);
#27769=VERTEX_POINT('',#92159);
#27770=VERTEX_POINT('',#92164);
#27771=VERTEX_POINT('',#92165);
#27772=VERTEX_POINT('',#92167);
#27773=VERTEX_POINT('',#92169);
#27774=VERTEX_POINT('',#92173);
#27775=VERTEX_POINT('',#92175);
#27776=VERTEX_POINT('',#92178);
#27777=VERTEX_POINT('',#92181);
#27778=VERTEX_POINT('',#92185);
#27779=VERTEX_POINT('',#92189);
#27780=VERTEX_POINT('',#92193);
#27781=VERTEX_POINT('',#92196);
#27782=VERTEX_POINT('',#92199);
#27783=VERTEX_POINT('',#92200);
#27784=VERTEX_POINT('',#92204);
#27785=VERTEX_POINT('',#92206);
#27786=VERTEX_POINT('',#92211);
#27787=VERTEX_POINT('',#92213);
#27788=VERTEX_POINT('',#92215);
#27789=VERTEX_POINT('',#92217);
#27790=VERTEX_POINT('',#92219);
#27791=VERTEX_POINT('',#92221);
#27792=VERTEX_POINT('',#92225);
#27793=VERTEX_POINT('',#92232);
#27794=VERTEX_POINT('',#92236);
#27795=VERTEX_POINT('',#92238);
#27796=VERTEX_POINT('',#92243);
#27797=VERTEX_POINT('',#92250);
#27798=VERTEX_POINT('',#92254);
#27799=VERTEX_POINT('',#92256);
#27800=VERTEX_POINT('',#92260);
#27801=VERTEX_POINT('',#92261);
#27802=VERTEX_POINT('',#92265);
#27803=VERTEX_POINT('',#92267);
#27804=VERTEX_POINT('',#92272);
#27805=VERTEX_POINT('',#92275);
#27806=VERTEX_POINT('',#92279);
#27807=VERTEX_POINT('',#92281);
#27808=VERTEX_POINT('',#92283);
#27809=VERTEX_POINT('',#92287);
#27810=VERTEX_POINT('',#92289);
#27811=VERTEX_POINT('',#92293);
#27812=VERTEX_POINT('',#92295);
#27813=VERTEX_POINT('',#92298);
#27814=VERTEX_POINT('',#92300);
#27815=VERTEX_POINT('',#92302);
#27816=VERTEX_POINT('',#92304);
#27817=VERTEX_POINT('',#92306);
#27818=VERTEX_POINT('',#92309);
#27819=VERTEX_POINT('',#92311);
#27820=VERTEX_POINT('',#92313);
#27821=VERTEX_POINT('',#92317);
#27822=VERTEX_POINT('',#92321);
#27823=VERTEX_POINT('',#92323);
#27824=VERTEX_POINT('',#92325);
#27825=VERTEX_POINT('',#92341);
#27826=VERTEX_POINT('',#92345);
#27827=VERTEX_POINT('',#92349);
#27828=VERTEX_POINT('',#92353);
#27829=VERTEX_POINT('',#92357);
#27830=VERTEX_POINT('',#92361);
#27831=VERTEX_POINT('',#92365);
#27832=VERTEX_POINT('',#92369);
#27833=VERTEX_POINT('',#92373);
#27834=VERTEX_POINT('',#92376);
#27835=VERTEX_POINT('',#92379);
#27836=VERTEX_POINT('',#92382);
#27837=VERTEX_POINT('',#92385);
#27838=VERTEX_POINT('',#92387);
#27839=VERTEX_POINT('',#92394);
#27840=VERTEX_POINT('',#92396);
#27841=VERTEX_POINT('',#92398);
#27842=VERTEX_POINT('',#92400);
#27843=VERTEX_POINT('',#92402);
#27844=VERTEX_POINT('',#92406);
#27845=VERTEX_POINT('',#92407);
#27846=VERTEX_POINT('',#92411);
#27847=VERTEX_POINT('',#92417);
#27848=VERTEX_POINT('',#92419);
#27849=VERTEX_POINT('',#92421);
#27850=VERTEX_POINT('',#92423);
#27851=VERTEX_POINT('',#92427);
#27852=VERTEX_POINT('',#92428);
#27853=VERTEX_POINT('',#92433);
#27854=VERTEX_POINT('',#92435);
#27855=VERTEX_POINT('',#92439);
#27856=VERTEX_POINT('',#92441);
#27857=VERTEX_POINT('',#92443);
#27858=VERTEX_POINT('',#92445);
#27859=VERTEX_POINT('',#92447);
#27860=VERTEX_POINT('',#92449);
#27861=VERTEX_POINT('',#92451);
#27862=VERTEX_POINT('',#92453);
#27863=VERTEX_POINT('',#92457);
#27864=VERTEX_POINT('',#92461);
#27865=VERTEX_POINT('',#92463);
#27866=VERTEX_POINT('',#92465);
#27867=VERTEX_POINT('',#92469);
#27868=VERTEX_POINT('',#92471);
#27869=VERTEX_POINT('',#92473);
#27870=VERTEX_POINT('',#92475);
#27871=VERTEX_POINT('',#92481);
#27872=VERTEX_POINT('',#92488);
#27873=VERTEX_POINT('',#92492);
#27874=VERTEX_POINT('',#92499);
#27875=VERTEX_POINT('',#92506);
#27876=VERTEX_POINT('',#92513);
#35080=EDGE_CURVE('',#27763,#27764,#14156,.T.);
#35081=EDGE_CURVE('',#27763,#27765,#1001,.T.);
#35082=EDGE_CURVE('',#27765,#27766,#142,.T.);
#35083=EDGE_CURVE('',#27766,#27764,#1002,.T.);
#35084=EDGE_CURVE('',#27767,#27768,#1003,.T.);
#35085=EDGE_CURVE('',#27768,#27769,#14157,.T.);
#35086=EDGE_CURVE('',#27769,#27769,#1004,.T.);
#35087=EDGE_CURVE('',#27768,#27767,#1005,.T.);
#35088=EDGE_CURVE('',#27770,#27771,#14158,.T.);
#35089=EDGE_CURVE('',#27772,#27770,#14159,.T.);
#35090=EDGE_CURVE('',#27773,#27772,#1006,.T.);
#35091=EDGE_CURVE('',#27772,#27773,#1007,.T.);
#35092=EDGE_CURVE('',#27767,#27772,#14160,.T.);
#35093=EDGE_CURVE('',#27774,#27767,#14161,.T.);
#35094=EDGE_CURVE('',#27775,#27774,#14162,.T.);
#35095=EDGE_CURVE('',#27771,#27775,#14163,.T.);
#35096=EDGE_CURVE('',#27776,#27776,#1008,.T.);
#35097=EDGE_CURVE('',#27769,#27777,#14164,.T.);
#35098=EDGE_CURVE('',#27777,#27777,#1009,.T.);
#35099=EDGE_CURVE('',#27773,#27778,#14165,.T.);
#35100=EDGE_CURVE('',#27778,#27778,#1010,.T.);
#35101=EDGE_CURVE('',#27778,#27779,#14166,.T.);
#35102=EDGE_CURVE('',#27779,#27779,#1011,.T.);
#35103=EDGE_CURVE('',#27780,#27777,#14167,.T.);
#35104=EDGE_CURVE('',#27781,#27779,#14168,.T.);
#35105=EDGE_CURVE('',#27782,#27783,#143,.T.);
#35106=EDGE_CURVE('',#27783,#27784,#1012,.T.);
#35107=EDGE_CURVE('',#27784,#27785,#14169,.T.);
#35108=EDGE_CURVE('',#27785,#27785,#1013,.T.);
#35109=EDGE_CURVE('',#27784,#27782,#1014,.T.);
#35110=EDGE_CURVE('',#27782,#27786,#14170,.T.);
#35111=EDGE_CURVE('',#27786,#27787,#14171,.T.);
#35112=EDGE_CURVE('',#27787,#27788,#14172,.T.);
#35113=EDGE_CURVE('',#27788,#27789,#14173,.T.);
#35114=EDGE_CURVE('',#27789,#27790,#14174,.T.);
#35115=EDGE_CURVE('',#27791,#27790,#144,.T.);
#35116=EDGE_CURVE('',#27791,#27792,#14175,.T.);
#35117=EDGE_CURVE('',#27766,#27792,#145,.T.);
#35118=EDGE_CURVE('',#27765,#27783,#14176,.T.);
#35119=EDGE_CURVE('',#27785,#27793,#14177,.T.);
#35120=EDGE_CURVE('',#27793,#27793,#595,.T.);
#35121=EDGE_CURVE('',#27790,#27794,#1015,.T.);
#35122=EDGE_CURVE('',#27794,#27795,#14178,.T.);
#35123=EDGE_CURVE('',#27795,#27795,#1016,.T.);
#35124=EDGE_CURVE('',#27794,#27791,#1017,.T.);
#35125=EDGE_CURVE('',#27795,#27796,#14179,.T.);
#35126=EDGE_CURVE('',#27796,#27796,#596,.T.);
#35127=EDGE_CURVE('',#27764,#27766,#1018,.T.);
#35128=EDGE_CURVE('',#27792,#27763,#1019,.T.);
#35129=EDGE_CURVE('',#27764,#27797,#14180,.T.);
#35130=EDGE_CURVE('',#27797,#27797,#597,.T.);
#35131=EDGE_CURVE('',#27798,#27789,#14181,.T.);
#35132=EDGE_CURVE('',#27799,#27798,#14182,.T.);
#35133=EDGE_CURVE('',#27786,#27799,#14183,.T.);
#35134=EDGE_CURVE('',#27800,#27801,#146,.T.);
#35135=EDGE_CURVE('',#27801,#27802,#1020,.T.);
#35136=EDGE_CURVE('',#27802,#27803,#14184,.T.);
#35137=EDGE_CURVE('',#27803,#27803,#1021,.T.);
#35138=EDGE_CURVE('',#27802,#27800,#1022,.T.);
#35139=EDGE_CURVE('',#27800,#27804,#14185,.T.);
#35140=EDGE_CURVE('',#27804,#27771,#14186,.T.);
#35141=EDGE_CURVE('',#27775,#27805,#14187,.T.);
#35142=EDGE_CURVE('',#27805,#27801,#14188,.T.);
#35143=EDGE_CURVE('',#27803,#27806,#14189,.T.);
#35144=EDGE_CURVE('',#27806,#27807,#1023,.T.);
#35145=EDGE_CURVE('',#27807,#27808,#1024,.T.);
#35146=EDGE_CURVE('',#27808,#27806,#1025,.T.);
#35147=EDGE_CURVE('',#27809,#27809,#1026,.T.);
#35148=EDGE_CURVE('',#27809,#27810,#14190,.T.);
#35149=EDGE_CURVE('',#27810,#27810,#1027,.T.);
#35150=EDGE_CURVE('',#27811,#27805,#14191,.T.);
#35151=EDGE_CURVE('',#27812,#27811,#14192,.T.);
#35152=EDGE_CURVE('',#27804,#27812,#14193,.T.);
#35153=EDGE_CURVE('',#27813,#27813,#1028,.T.);
#35154=EDGE_CURVE('',#27814,#27814,#1029,.T.);
#35155=EDGE_CURVE('',#27815,#27815,#1030,.T.);
#35156=EDGE_CURVE('',#27816,#27816,#1031,.T.);
#35157=EDGE_CURVE('',#27817,#27817,#1032,.T.);
#35158=EDGE_CURVE('',#27810,#27818,#14194,.T.);
#35159=EDGE_CURVE('',#27818,#27819,#1033,.T.);
#35160=EDGE_CURVE('',#27819,#27820,#1034,.T.);
#35161=EDGE_CURVE('',#27820,#27818,#1035,.T.);
#35162=EDGE_CURVE('',#27813,#27821,#14195,.T.);
#35163=EDGE_CURVE('',#27821,#27821,#1036,.T.);
#35164=EDGE_CURVE('',#27821,#27822,#14196,.T.);
#35165=EDGE_CURVE('',#27822,#27823,#1037,.T.);
#35166=EDGE_CURVE('',#27823,#27824,#1038,.T.);
#35167=EDGE_CURVE('',#27824,#27822,#1039,.T.);
#35168=EDGE_CURVE('',#27823,#27824,#14197,.T.);
#35169=EDGE_CURVE('',#27823,#27824,#14198,.T.);
#35170=EDGE_CURVE('',#27819,#27820,#14199,.T.);
#35171=EDGE_CURVE('',#27819,#27820,#14200,.T.);
#35172=EDGE_CURVE('',#27807,#27808,#14201,.T.);
#35173=EDGE_CURVE('',#27807,#27808,#14202,.T.);
#35174=EDGE_CURVE('',#27814,#27825,#14203,.T.);
#35175=EDGE_CURVE('',#27825,#27825,#1040,.T.);
#35176=EDGE_CURVE('',#27825,#27826,#14204,.T.);
#35177=EDGE_CURVE('',#27826,#27826,#1041,.T.);
#35178=EDGE_CURVE('',#27817,#27827,#14205,.T.);
#35179=EDGE_CURVE('',#27827,#27827,#1042,.T.);
#35180=EDGE_CURVE('',#27827,#27828,#14206,.T.);
#35181=EDGE_CURVE('',#27828,#27828,#1043,.T.);
#35182=EDGE_CURVE('',#27815,#27829,#14207,.T.);
#35183=EDGE_CURVE('',#27829,#27829,#1044,.T.);
#35184=EDGE_CURVE('',#27829,#27830,#14208,.T.);
#35185=EDGE_CURVE('',#27830,#27830,#1045,.T.);
#35186=EDGE_CURVE('',#27816,#27831,#14209,.T.);
#35187=EDGE_CURVE('',#27831,#27831,#1046,.T.);
#35188=EDGE_CURVE('',#27831,#27832,#14210,.T.);
#35189=EDGE_CURVE('',#27832,#27832,#1047,.T.);
#35190=EDGE_CURVE('',#27826,#27833,#14211,.T.);
#35191=EDGE_CURVE('',#27832,#27834,#14212,.T.);
#35192=EDGE_CURVE('',#27830,#27835,#14213,.T.);
#35193=EDGE_CURVE('',#27828,#27836,#14214,.T.);
#35194=EDGE_CURVE('',#27776,#27837,#14215,.T.);
#35195=EDGE_CURVE('',#27837,#27838,#1048,.T.);
#35196=EDGE_CURVE('',#27838,#27837,#1049,.T.);
#35197=EDGE_CURVE('',#27838,#27808,#14216,.T.);
#35198=EDGE_CURVE('',#27807,#27820,#14217,.T.);
#35199=EDGE_CURVE('',#27819,#27824,#14218,.T.);
#35200=EDGE_CURVE('',#27823,#27839,#14219,.T.);
#35201=EDGE_CURVE('',#27839,#27840,#1050,.T.);
#35202=EDGE_CURVE('',#27841,#27840,#14220,.T.);
#35203=EDGE_CURVE('',#27842,#27841,#1051,.T.);
#35204=EDGE_CURVE('',#27843,#27842,#14221,.T.);
#35205=EDGE_CURVE('',#27843,#27839,#1052,.T.);
#35206=EDGE_CURVE('',#27844,#27845,#14222,.T.);
#35207=EDGE_CURVE('',#27845,#27845,#1053,.T.);
#35208=EDGE_CURVE('',#27846,#27846,#1054,.T.);
#35209=EDGE_CURVE('',#27846,#27845,#14223,.T.);
#35210=EDGE_CURVE('',#27840,#27843,#14224,.T.);
#35211=EDGE_CURVE('',#27847,#27842,#14225,.T.);
#35212=EDGE_CURVE('',#27848,#27847,#14226,.T.);
#35213=EDGE_CURVE('',#27848,#27849,#14227,.T.);
#35214=EDGE_CURVE('',#27850,#27849,#14228,.T.);
#35215=EDGE_CURVE('',#27841,#27850,#14229,.T.);
#35216=EDGE_CURVE('',#27851,#27852,#14230,.T.);
#35217=EDGE_CURVE('',#27849,#27851,#14231,.T.);
#35218=EDGE_CURVE('',#27852,#27848,#14232,.T.);
#35219=EDGE_CURVE('',#27853,#27850,#14233,.T.);
#35220=EDGE_CURVE('',#27854,#27853,#14234,.T.);
#35221=EDGE_CURVE('',#27847,#27854,#14235,.T.);
#35222=EDGE_CURVE('',#27854,#27855,#14236,.T.);
#35223=EDGE_CURVE('',#27855,#27856,#14237,.T.);
#35224=EDGE_CURVE('',#27857,#27856,#14238,.T.);
#35225=EDGE_CURVE('',#27858,#27857,#14239,.T.);
#35226=EDGE_CURVE('',#27859,#27858,#14240,.T.);
#35227=EDGE_CURVE('',#27860,#27859,#14241,.T.);
#35228=EDGE_CURVE('',#27861,#27860,#14242,.T.);
#35229=EDGE_CURVE('',#27861,#27862,#14243,.T.);
#35230=EDGE_CURVE('',#27862,#27852,#14244,.T.);
#35231=EDGE_CURVE('',#27863,#27853,#14245,.T.);
#35232=EDGE_CURVE('',#27855,#27863,#14246,.T.);
#35233=EDGE_CURVE('',#27856,#27864,#14247,.T.);
#35234=EDGE_CURVE('',#27865,#27863,#14248,.T.);
#35235=EDGE_CURVE('',#27866,#27865,#14249,.T.);
#35236=EDGE_CURVE('',#27864,#27866,#14250,.T.);
#35237=EDGE_CURVE('',#27867,#27861,#14251,.T.);
#35238=EDGE_CURVE('',#27868,#27867,#14252,.T.);
#35239=EDGE_CURVE('',#27869,#27868,#14253,.T.);
#35240=EDGE_CURVE('',#27870,#27869,#14254,.T.);
#35241=EDGE_CURVE('',#27862,#27870,#14255,.T.);
#35242=EDGE_CURVE('',#27851,#27870,#14256,.T.);
#35243=EDGE_CURVE('',#27864,#27871,#14257,.T.);
#35244=EDGE_CURVE('',#27871,#27857,#14258,.T.);
#35245=EDGE_CURVE('',#27860,#27788,#14259,.T.);
#35246=EDGE_CURVE('',#27788,#27867,#14260,.T.);
#35247=EDGE_CURVE('',#27872,#27866,#14261,.T.);
#35248=EDGE_CURVE('',#27871,#27872,#14262,.T.);
#35249=EDGE_CURVE('',#27865,#27873,#14263,.T.);
#35250=EDGE_CURVE('',#27873,#27872,#14264,.T.);
#35251=EDGE_CURVE('',#27774,#27873,#14265,.T.);
#35252=EDGE_CURVE('',#27872,#27774,#14266,.T.);
#35253=EDGE_CURVE('',#27805,#27874,#14267,.T.);
#35254=EDGE_CURVE('',#27874,#27775,#14268,.T.);
#35255=EDGE_CURVE('',#27770,#27871,#14269,.T.);
#35256=EDGE_CURVE('',#27857,#27770,#14270,.T.);
#35257=EDGE_CURVE('',#27787,#27875,#14271,.T.);
#35258=EDGE_CURVE('',#27875,#27786,#14272,.T.);
#35259=EDGE_CURVE('',#27858,#27804,#14273,.T.);
#35260=EDGE_CURVE('',#27771,#27858,#14274,.T.);
#35261=EDGE_CURVE('',#27799,#27876,#14275,.T.);
#35262=EDGE_CURVE('',#27811,#27799,#14276,.T.);
#35263=EDGE_CURVE('',#27876,#27811,#14277,.T.);
#35264=EDGE_CURVE('',#27789,#27860,#14278,.T.);
#35265=EDGE_CURVE('',#27859,#27798,#14279,.T.);
#35266=EDGE_CURVE('',#27812,#27859,#14280,.T.);
#35267=EDGE_CURVE('',#27798,#27812,#14281,.T.);
#35268=EDGE_CURVE('',#27874,#27876,#14282,.T.);
#35269=EDGE_CURVE('',#27876,#27875,#14283,.T.);
#35270=EDGE_CURVE('',#27868,#27787,#14284,.T.);
#35271=EDGE_CURVE('',#27875,#27869,#14285,.T.);
#35272=EDGE_CURVE('',#27873,#27874,#14286,.T.);
#48495=ORIENTED_EDGE('',*,*,#35080,.F.);
#48496=ORIENTED_EDGE('',*,*,#35081,.T.);
#48497=ORIENTED_EDGE('',*,*,#35082,.T.);
#48498=ORIENTED_EDGE('',*,*,#35083,.T.);
#48499=ORIENTED_EDGE('',*,*,#35084,.T.);
#48500=ORIENTED_EDGE('',*,*,#35085,.T.);
#48501=ORIENTED_EDGE('',*,*,#35086,.T.);
#48502=ORIENTED_EDGE('',*,*,#35085,.F.);
#48503=ORIENTED_EDGE('',*,*,#35087,.T.);
#48504=ORIENTED_EDGE('',*,*,#35088,.F.);
#48505=ORIENTED_EDGE('',*,*,#35089,.F.);
#48506=ORIENTED_EDGE('',*,*,#35090,.F.);
#48507=ORIENTED_EDGE('',*,*,#35091,.F.);
#48508=ORIENTED_EDGE('',*,*,#35092,.F.);
#48509=ORIENTED_EDGE('',*,*,#35087,.F.);
#48510=ORIENTED_EDGE('',*,*,#35084,.F.);
#48511=ORIENTED_EDGE('',*,*,#35093,.F.);
#48512=ORIENTED_EDGE('',*,*,#35094,.F.);
#48513=ORIENTED_EDGE('',*,*,#35095,.F.);
#48514=ORIENTED_EDGE('',*,*,#35096,.F.);
#48515=ORIENTED_EDGE('',*,*,#35086,.F.);
#48516=ORIENTED_EDGE('',*,*,#35097,.T.);
#48517=ORIENTED_EDGE('',*,*,#35098,.T.);
#48518=ORIENTED_EDGE('',*,*,#35097,.F.);
#48519=ORIENTED_EDGE('',*,*,#35091,.T.);
#48520=ORIENTED_EDGE('',*,*,#35099,.T.);
#48521=ORIENTED_EDGE('',*,*,#35100,.T.);
#48522=ORIENTED_EDGE('',*,*,#35099,.F.);
#48523=ORIENTED_EDGE('',*,*,#35090,.T.);
#48524=ORIENTED_EDGE('',*,*,#35100,.F.);
#48525=ORIENTED_EDGE('',*,*,#35101,.T.);
#48526=ORIENTED_EDGE('',*,*,#35102,.T.);
#48527=ORIENTED_EDGE('',*,*,#35101,.F.);
#48528=ORIENTED_EDGE('',*,*,#35103,.T.);
#48529=ORIENTED_EDGE('',*,*,#35098,.F.);
#48530=ORIENTED_EDGE('',*,*,#35103,.F.);
#48531=ORIENTED_EDGE('',*,*,#35104,.T.);
#48532=ORIENTED_EDGE('',*,*,#35102,.F.);
#48533=ORIENTED_EDGE('',*,*,#35104,.F.);
#48534=ORIENTED_EDGE('',*,*,#35105,.T.);
#48535=ORIENTED_EDGE('',*,*,#35106,.T.);
#48536=ORIENTED_EDGE('',*,*,#35107,.T.);
#48537=ORIENTED_EDGE('',*,*,#35108,.T.);
#48538=ORIENTED_EDGE('',*,*,#35107,.F.);
#48539=ORIENTED_EDGE('',*,*,#35109,.T.);
#48540=ORIENTED_EDGE('',*,*,#35105,.F.);
#48541=ORIENTED_EDGE('',*,*,#35110,.T.);
#48542=ORIENTED_EDGE('',*,*,#35111,.T.);
#48543=ORIENTED_EDGE('',*,*,#35112,.T.);
#48544=ORIENTED_EDGE('',*,*,#35113,.T.);
#48545=ORIENTED_EDGE('',*,*,#35114,.T.);
#48546=ORIENTED_EDGE('',*,*,#35115,.F.);
#48547=ORIENTED_EDGE('',*,*,#35116,.T.);
#48548=ORIENTED_EDGE('',*,*,#35117,.F.);
#48549=ORIENTED_EDGE('',*,*,#35082,.F.);
#48550=ORIENTED_EDGE('',*,*,#35118,.T.);
#48551=ORIENTED_EDGE('',*,*,#35108,.F.);
#48552=ORIENTED_EDGE('',*,*,#35119,.T.);
#48553=ORIENTED_EDGE('',*,*,#35120,.F.);
#48554=ORIENTED_EDGE('',*,*,#35119,.F.);
#48555=ORIENTED_EDGE('',*,*,#35115,.T.);
#48556=ORIENTED_EDGE('',*,*,#35121,.T.);
#48557=ORIENTED_EDGE('',*,*,#35122,.T.);
#48558=ORIENTED_EDGE('',*,*,#35123,.T.);
#48559=ORIENTED_EDGE('',*,*,#35122,.F.);
#48560=ORIENTED_EDGE('',*,*,#35124,.T.);
#48561=ORIENTED_EDGE('',*,*,#35123,.F.);
#48562=ORIENTED_EDGE('',*,*,#35125,.T.);
#48563=ORIENTED_EDGE('',*,*,#35126,.F.);
#48564=ORIENTED_EDGE('',*,*,#35125,.F.);
#48565=ORIENTED_EDGE('',*,*,#35080,.T.);
#48566=ORIENTED_EDGE('',*,*,#35127,.T.);
#48567=ORIENTED_EDGE('',*,*,#35117,.T.);
#48568=ORIENTED_EDGE('',*,*,#35128,.T.);
#48569=ORIENTED_EDGE('',*,*,#35083,.F.);
#48570=ORIENTED_EDGE('',*,*,#35127,.F.);
#48571=ORIENTED_EDGE('',*,*,#35129,.T.);
#48572=ORIENTED_EDGE('',*,*,#35130,.F.);
#48573=ORIENTED_EDGE('',*,*,#35129,.F.);
#48574=ORIENTED_EDGE('',*,*,#35106,.F.);
#48575=ORIENTED_EDGE('',*,*,#35118,.F.);
#48576=ORIENTED_EDGE('',*,*,#35081,.F.);
#48577=ORIENTED_EDGE('',*,*,#35128,.F.);
#48578=ORIENTED_EDGE('',*,*,#35116,.F.);
#48579=ORIENTED_EDGE('',*,*,#35124,.F.);
#48580=ORIENTED_EDGE('',*,*,#35121,.F.);
#48581=ORIENTED_EDGE('',*,*,#35114,.F.);
#48582=ORIENTED_EDGE('',*,*,#35131,.F.);
#48583=ORIENTED_EDGE('',*,*,#35132,.F.);
#48584=ORIENTED_EDGE('',*,*,#35133,.F.);
#48585=ORIENTED_EDGE('',*,*,#35110,.F.);
#48586=ORIENTED_EDGE('',*,*,#35109,.F.);
#48587=ORIENTED_EDGE('',*,*,#35134,.T.);
#48588=ORIENTED_EDGE('',*,*,#35135,.T.);
#48589=ORIENTED_EDGE('',*,*,#35136,.T.);
#48590=ORIENTED_EDGE('',*,*,#35137,.T.);
#48591=ORIENTED_EDGE('',*,*,#35136,.F.);
#48592=ORIENTED_EDGE('',*,*,#35138,.T.);
#48593=ORIENTED_EDGE('',*,*,#35134,.F.);
#48594=ORIENTED_EDGE('',*,*,#35139,.T.);
#48595=ORIENTED_EDGE('',*,*,#35140,.T.);
#48596=ORIENTED_EDGE('',*,*,#35095,.T.);
#48597=ORIENTED_EDGE('',*,*,#35141,.T.);
#48598=ORIENTED_EDGE('',*,*,#35142,.T.);
#48599=ORIENTED_EDGE('',*,*,#35137,.F.);
#48600=ORIENTED_EDGE('',*,*,#35143,.T.);
#48601=ORIENTED_EDGE('',*,*,#35144,.T.);
#48602=ORIENTED_EDGE('',*,*,#35145,.T.);
#48603=ORIENTED_EDGE('',*,*,#35146,.T.);
#48604=ORIENTED_EDGE('',*,*,#35143,.F.);
#48605=ORIENTED_EDGE('',*,*,#35147,.T.);
#48606=ORIENTED_EDGE('',*,*,#35148,.T.);
#48607=ORIENTED_EDGE('',*,*,#35149,.T.);
#48608=ORIENTED_EDGE('',*,*,#35148,.F.);
#48609=ORIENTED_EDGE('',*,*,#35135,.F.);
#48610=ORIENTED_EDGE('',*,*,#35142,.F.);
#48611=ORIENTED_EDGE('',*,*,#35150,.F.);
#48612=ORIENTED_EDGE('',*,*,#35151,.F.);
#48613=ORIENTED_EDGE('',*,*,#35152,.F.);
#48614=ORIENTED_EDGE('',*,*,#35139,.F.);
#48615=ORIENTED_EDGE('',*,*,#35138,.F.);
#48616=ORIENTED_EDGE('',*,*,#35153,.F.);
#48617=ORIENTED_EDGE('',*,*,#35154,.F.);
#48618=ORIENTED_EDGE('',*,*,#35155,.F.);
#48619=ORIENTED_EDGE('',*,*,#35156,.F.);
#48620=ORIENTED_EDGE('',*,*,#35157,.F.);
#48621=ORIENTED_EDGE('',*,*,#35147,.F.);
#48622=ORIENTED_EDGE('',*,*,#35149,.F.);
#48623=ORIENTED_EDGE('',*,*,#35158,.T.);
#48624=ORIENTED_EDGE('',*,*,#35159,.T.);
#48625=ORIENTED_EDGE('',*,*,#35160,.T.);
#48626=ORIENTED_EDGE('',*,*,#35161,.T.);
#48627=ORIENTED_EDGE('',*,*,#35158,.F.);
#48628=ORIENTED_EDGE('',*,*,#35153,.T.);
#48629=ORIENTED_EDGE('',*,*,#35162,.T.);
#48630=ORIENTED_EDGE('',*,*,#35163,.T.);
#48631=ORIENTED_EDGE('',*,*,#35162,.F.);
#48632=ORIENTED_EDGE('',*,*,#35163,.F.);
#48633=ORIENTED_EDGE('',*,*,#35164,.T.);
#48634=ORIENTED_EDGE('',*,*,#35165,.T.);
#48635=ORIENTED_EDGE('',*,*,#35166,.T.);
#48636=ORIENTED_EDGE('',*,*,#35167,.T.);
#48637=ORIENTED_EDGE('',*,*,#35164,.F.);
#48638=ORIENTED_EDGE('',*,*,#35168,.T.);
#48639=ORIENTED_EDGE('',*,*,#35166,.F.);
#48640=ORIENTED_EDGE('',*,*,#35169,.F.);
#48641=ORIENTED_EDGE('',*,*,#35165,.F.);
#48642=ORIENTED_EDGE('',*,*,#35167,.F.);
#48643=ORIENTED_EDGE('',*,*,#35170,.T.);
#48644=ORIENTED_EDGE('',*,*,#35160,.F.);
#48645=ORIENTED_EDGE('',*,*,#35171,.F.);
#48646=ORIENTED_EDGE('',*,*,#35159,.F.);
#48647=ORIENTED_EDGE('',*,*,#35161,.F.);
#48648=ORIENTED_EDGE('',*,*,#35172,.T.);
#48649=ORIENTED_EDGE('',*,*,#35145,.F.);
#48650=ORIENTED_EDGE('',*,*,#35173,.F.);
#48651=ORIENTED_EDGE('',*,*,#35144,.F.);
#48652=ORIENTED_EDGE('',*,*,#35146,.F.);
#48653=ORIENTED_EDGE('',*,*,#35154,.T.);
#48654=ORIENTED_EDGE('',*,*,#35174,.T.);
#48655=ORIENTED_EDGE('',*,*,#35175,.T.);
#48656=ORIENTED_EDGE('',*,*,#35174,.F.);
#48657=ORIENTED_EDGE('',*,*,#35175,.F.);
#48658=ORIENTED_EDGE('',*,*,#35176,.T.);
#48659=ORIENTED_EDGE('',*,*,#35177,.T.);
#48660=ORIENTED_EDGE('',*,*,#35176,.F.);
#48661=ORIENTED_EDGE('',*,*,#35157,.T.);
#48662=ORIENTED_EDGE('',*,*,#35178,.T.);
#48663=ORIENTED_EDGE('',*,*,#35179,.T.);
#48664=ORIENTED_EDGE('',*,*,#35178,.F.);
#48665=ORIENTED_EDGE('',*,*,#35179,.F.);
#48666=ORIENTED_EDGE('',*,*,#35180,.T.);
#48667=ORIENTED_EDGE('',*,*,#35181,.T.);
#48668=ORIENTED_EDGE('',*,*,#35180,.F.);
#48669=ORIENTED_EDGE('',*,*,#35155,.T.);
#48670=ORIENTED_EDGE('',*,*,#35182,.T.);
#48671=ORIENTED_EDGE('',*,*,#35183,.T.);
#48672=ORIENTED_EDGE('',*,*,#35182,.F.);
#48673=ORIENTED_EDGE('',*,*,#35183,.F.);
#48674=ORIENTED_EDGE('',*,*,#35184,.T.);
#48675=ORIENTED_EDGE('',*,*,#35185,.T.);
#48676=ORIENTED_EDGE('',*,*,#35184,.F.);
#48677=ORIENTED_EDGE('',*,*,#35156,.T.);
#48678=ORIENTED_EDGE('',*,*,#35186,.T.);
#48679=ORIENTED_EDGE('',*,*,#35187,.T.);
#48680=ORIENTED_EDGE('',*,*,#35186,.F.);
#48681=ORIENTED_EDGE('',*,*,#35187,.F.);
#48682=ORIENTED_EDGE('',*,*,#35188,.T.);
#48683=ORIENTED_EDGE('',*,*,#35189,.T.);
#48684=ORIENTED_EDGE('',*,*,#35188,.F.);
#48685=ORIENTED_EDGE('',*,*,#35177,.F.);
#48686=ORIENTED_EDGE('',*,*,#35190,.T.);
#48687=ORIENTED_EDGE('',*,*,#35190,.F.);
#48688=ORIENTED_EDGE('',*,*,#35189,.F.);
#48689=ORIENTED_EDGE('',*,*,#35191,.T.);
#48690=ORIENTED_EDGE('',*,*,#35191,.F.);
#48691=ORIENTED_EDGE('',*,*,#35185,.F.);
#48692=ORIENTED_EDGE('',*,*,#35192,.T.);
#48693=ORIENTED_EDGE('',*,*,#35192,.F.);
#48694=ORIENTED_EDGE('',*,*,#35181,.F.);
#48695=ORIENTED_EDGE('',*,*,#35193,.T.);
#48696=ORIENTED_EDGE('',*,*,#35193,.F.);
#48697=ORIENTED_EDGE('',*,*,#35096,.T.);
#48698=ORIENTED_EDGE('',*,*,#35194,.T.);
#48699=ORIENTED_EDGE('',*,*,#35195,.T.);
#48700=ORIENTED_EDGE('',*,*,#35196,.T.);
#48701=ORIENTED_EDGE('',*,*,#35194,.F.);
#48702=ORIENTED_EDGE('',*,*,#35195,.F.);
#48703=ORIENTED_EDGE('',*,*,#35196,.F.);
#48704=ORIENTED_EDGE('',*,*,#35197,.T.);
#48705=ORIENTED_EDGE('',*,*,#35172,.F.);
#48706=ORIENTED_EDGE('',*,*,#35198,.T.);
#48707=ORIENTED_EDGE('',*,*,#35170,.F.);
#48708=ORIENTED_EDGE('',*,*,#35199,.T.);
#48709=ORIENTED_EDGE('',*,*,#35168,.F.);
#48710=ORIENTED_EDGE('',*,*,#35200,.T.);
#48711=ORIENTED_EDGE('',*,*,#35201,.T.);
#48712=ORIENTED_EDGE('',*,*,#35202,.F.);
#48713=ORIENTED_EDGE('',*,*,#35203,.F.);
#48714=ORIENTED_EDGE('',*,*,#35204,.F.);
#48715=ORIENTED_EDGE('',*,*,#35205,.T.);
#48716=ORIENTED_EDGE('',*,*,#35200,.F.);
#48717=ORIENTED_EDGE('',*,*,#35169,.T.);
#48718=ORIENTED_EDGE('',*,*,#35199,.F.);
#48719=ORIENTED_EDGE('',*,*,#35171,.T.);
#48720=ORIENTED_EDGE('',*,*,#35198,.F.);
#48721=ORIENTED_EDGE('',*,*,#35173,.T.);
#48722=ORIENTED_EDGE('',*,*,#35197,.F.);
#48723=ORIENTED_EDGE('',*,*,#35206,.T.);
#48724=ORIENTED_EDGE('',*,*,#35207,.F.);
#48725=ORIENTED_EDGE('',*,*,#35206,.F.);
#48726=ORIENTED_EDGE('',*,*,#35208,.F.);
#48727=ORIENTED_EDGE('',*,*,#35209,.T.);
#48728=ORIENTED_EDGE('',*,*,#35207,.T.);
#48729=ORIENTED_EDGE('',*,*,#35209,.F.);
#48730=ORIENTED_EDGE('',*,*,#35210,.F.);
#48731=ORIENTED_EDGE('',*,*,#35201,.F.);
#48732=ORIENTED_EDGE('',*,*,#35205,.F.);
#48733=ORIENTED_EDGE('',*,*,#35208,.T.);
#48734=ORIENTED_EDGE('',*,*,#35202,.T.);
#48735=ORIENTED_EDGE('',*,*,#35210,.T.);
#48736=ORIENTED_EDGE('',*,*,#35204,.T.);
#48737=ORIENTED_EDGE('',*,*,#35211,.F.);
#48738=ORIENTED_EDGE('',*,*,#35212,.F.);
#48739=ORIENTED_EDGE('',*,*,#35213,.T.);
#48740=ORIENTED_EDGE('',*,*,#35214,.F.);
#48741=ORIENTED_EDGE('',*,*,#35215,.F.);
#48742=ORIENTED_EDGE('',*,*,#35216,.F.);
#48743=ORIENTED_EDGE('',*,*,#35217,.F.);
#48744=ORIENTED_EDGE('',*,*,#35213,.F.);
#48745=ORIENTED_EDGE('',*,*,#35218,.F.);
#48746=ORIENTED_EDGE('',*,*,#35203,.T.);
#48747=ORIENTED_EDGE('',*,*,#35215,.T.);
#48748=ORIENTED_EDGE('',*,*,#35219,.F.);
#48749=ORIENTED_EDGE('',*,*,#35220,.F.);
#48750=ORIENTED_EDGE('',*,*,#35221,.F.);
#48751=ORIENTED_EDGE('',*,*,#35211,.T.);
#48752=ORIENTED_EDGE('',*,*,#35218,.T.);
#48753=ORIENTED_EDGE('',*,*,#35212,.T.);
#48754=ORIENTED_EDGE('',*,*,#35221,.T.);
#48755=ORIENTED_EDGE('',*,*,#35222,.T.);
#48756=ORIENTED_EDGE('',*,*,#35223,.T.);
#48757=ORIENTED_EDGE('',*,*,#35224,.F.);
#48758=ORIENTED_EDGE('',*,*,#35225,.F.);
#48759=ORIENTED_EDGE('',*,*,#35226,.F.);
#48760=ORIENTED_EDGE('',*,*,#35227,.F.);
#48761=ORIENTED_EDGE('',*,*,#35228,.F.);
#48762=ORIENTED_EDGE('',*,*,#35229,.T.);
#48763=ORIENTED_EDGE('',*,*,#35230,.T.);
#48764=ORIENTED_EDGE('',*,*,#35220,.T.);
#48765=ORIENTED_EDGE('',*,*,#35231,.F.);
#48766=ORIENTED_EDGE('',*,*,#35232,.F.);
#48767=ORIENTED_EDGE('',*,*,#35222,.F.);
#48768=ORIENTED_EDGE('',*,*,#35233,.F.);
#48769=ORIENTED_EDGE('',*,*,#35223,.F.);
#48770=ORIENTED_EDGE('',*,*,#35232,.T.);
#48771=ORIENTED_EDGE('',*,*,#35234,.F.);
#48772=ORIENTED_EDGE('',*,*,#35235,.F.);
#48773=ORIENTED_EDGE('',*,*,#35236,.F.);
#48774=ORIENTED_EDGE('',*,*,#35237,.F.);
#48775=ORIENTED_EDGE('',*,*,#35238,.F.);
#48776=ORIENTED_EDGE('',*,*,#35239,.F.);
#48777=ORIENTED_EDGE('',*,*,#35240,.F.);
#48778=ORIENTED_EDGE('',*,*,#35241,.F.);
#48779=ORIENTED_EDGE('',*,*,#35229,.F.);
#48780=ORIENTED_EDGE('',*,*,#35126,.T.);
#48781=ORIENTED_EDGE('',*,*,#35120,.T.);
#48782=ORIENTED_EDGE('',*,*,#35130,.T.);
#48783=ORIENTED_EDGE('',*,*,#35216,.T.);
#48784=ORIENTED_EDGE('',*,*,#35230,.F.);
#48785=ORIENTED_EDGE('',*,*,#35241,.T.);
#48786=ORIENTED_EDGE('',*,*,#35242,.F.);
#48787=ORIENTED_EDGE('',*,*,#35233,.T.);
#48788=ORIENTED_EDGE('',*,*,#35243,.T.);
#48789=ORIENTED_EDGE('',*,*,#35244,.T.);
#48790=ORIENTED_EDGE('',*,*,#35224,.T.);
#48791=ORIENTED_EDGE('',*,*,#35237,.T.);
#48792=ORIENTED_EDGE('',*,*,#35228,.T.);
#48793=ORIENTED_EDGE('',*,*,#35245,.T.);
#48794=ORIENTED_EDGE('',*,*,#35246,.T.);
#48795=ORIENTED_EDGE('',*,*,#35236,.T.);
#48796=ORIENTED_EDGE('',*,*,#35247,.F.);
#48797=ORIENTED_EDGE('',*,*,#35248,.F.);
#48798=ORIENTED_EDGE('',*,*,#35243,.F.);
#48799=ORIENTED_EDGE('',*,*,#35235,.T.);
#48800=ORIENTED_EDGE('',*,*,#35249,.T.);
#48801=ORIENTED_EDGE('',*,*,#35250,.T.);
#48802=ORIENTED_EDGE('',*,*,#35247,.T.);
#48803=ORIENTED_EDGE('',*,*,#35251,.F.);
#48804=ORIENTED_EDGE('',*,*,#35252,.F.);
#48805=ORIENTED_EDGE('',*,*,#35250,.F.);
#48806=ORIENTED_EDGE('',*,*,#35253,.F.);
#48807=ORIENTED_EDGE('',*,*,#35141,.F.);
#48808=ORIENTED_EDGE('',*,*,#35254,.F.);
#48809=ORIENTED_EDGE('',*,*,#35255,.F.);
#48810=ORIENTED_EDGE('',*,*,#35256,.F.);
#48811=ORIENTED_EDGE('',*,*,#35244,.F.);
#48812=ORIENTED_EDGE('',*,*,#35257,.F.);
#48813=ORIENTED_EDGE('',*,*,#35111,.F.);
#48814=ORIENTED_EDGE('',*,*,#35258,.F.);
#48815=ORIENTED_EDGE('',*,*,#35140,.F.);
#48816=ORIENTED_EDGE('',*,*,#35259,.F.);
#48817=ORIENTED_EDGE('',*,*,#35260,.F.);
#48818=ORIENTED_EDGE('',*,*,#35261,.F.);
#48819=ORIENTED_EDGE('',*,*,#35262,.F.);
#48820=ORIENTED_EDGE('',*,*,#35263,.F.);
#48821=ORIENTED_EDGE('',*,*,#35113,.F.);
#48822=ORIENTED_EDGE('',*,*,#35245,.F.);
#48823=ORIENTED_EDGE('',*,*,#35264,.F.);
#48824=ORIENTED_EDGE('',*,*,#35265,.F.);
#48825=ORIENTED_EDGE('',*,*,#35266,.F.);
#48826=ORIENTED_EDGE('',*,*,#35267,.F.);
#48827=ORIENTED_EDGE('',*,*,#35266,.T.);
#48828=ORIENTED_EDGE('',*,*,#35226,.T.);
#48829=ORIENTED_EDGE('',*,*,#35259,.T.);
#48830=ORIENTED_EDGE('',*,*,#35152,.T.);
#48831=ORIENTED_EDGE('',*,*,#35262,.T.);
#48832=ORIENTED_EDGE('',*,*,#35132,.T.);
#48833=ORIENTED_EDGE('',*,*,#35267,.T.);
#48834=ORIENTED_EDGE('',*,*,#35151,.T.);
#48835=ORIENTED_EDGE('',*,*,#35264,.T.);
#48836=ORIENTED_EDGE('',*,*,#35227,.T.);
#48837=ORIENTED_EDGE('',*,*,#35265,.T.);
#48838=ORIENTED_EDGE('',*,*,#35131,.T.);
#48839=ORIENTED_EDGE('',*,*,#35253,.T.);
#48840=ORIENTED_EDGE('',*,*,#35268,.T.);
#48841=ORIENTED_EDGE('',*,*,#35263,.T.);
#48842=ORIENTED_EDGE('',*,*,#35150,.T.);
#48843=ORIENTED_EDGE('',*,*,#35261,.T.);
#48844=ORIENTED_EDGE('',*,*,#35269,.T.);
#48845=ORIENTED_EDGE('',*,*,#35258,.T.);
#48846=ORIENTED_EDGE('',*,*,#35133,.T.);
#48847=ORIENTED_EDGE('',*,*,#35260,.T.);
#48848=ORIENTED_EDGE('',*,*,#35225,.T.);
#48849=ORIENTED_EDGE('',*,*,#35256,.T.);
#48850=ORIENTED_EDGE('',*,*,#35088,.T.);
#48851=ORIENTED_EDGE('',*,*,#35239,.T.);
#48852=ORIENTED_EDGE('',*,*,#35270,.T.);
#48853=ORIENTED_EDGE('',*,*,#35257,.T.);
#48854=ORIENTED_EDGE('',*,*,#35271,.T.);
#48855=ORIENTED_EDGE('',*,*,#35252,.T.);
#48856=ORIENTED_EDGE('',*,*,#35093,.T.);
#48857=ORIENTED_EDGE('',*,*,#35092,.T.);
#48858=ORIENTED_EDGE('',*,*,#35089,.T.);
#48859=ORIENTED_EDGE('',*,*,#35255,.T.);
#48860=ORIENTED_EDGE('',*,*,#35248,.T.);
#48861=ORIENTED_EDGE('',*,*,#35251,.T.);
#48862=ORIENTED_EDGE('',*,*,#35272,.T.);
#48863=ORIENTED_EDGE('',*,*,#35254,.T.);
#48864=ORIENTED_EDGE('',*,*,#35094,.T.);
#48865=ORIENTED_EDGE('',*,*,#35238,.T.);
#48866=ORIENTED_EDGE('',*,*,#35246,.F.);
#48867=ORIENTED_EDGE('',*,*,#35112,.F.);
#48868=ORIENTED_EDGE('',*,*,#35270,.F.);
#48869=ORIENTED_EDGE('',*,*,#35217,.T.);
#48870=ORIENTED_EDGE('',*,*,#35242,.T.);
#48871=ORIENTED_EDGE('',*,*,#35240,.T.);
#48872=ORIENTED_EDGE('',*,*,#35271,.F.);
#48873=ORIENTED_EDGE('',*,*,#35269,.F.);
#48874=ORIENTED_EDGE('',*,*,#35268,.F.);
#48875=ORIENTED_EDGE('',*,*,#35272,.F.);
#48876=ORIENTED_EDGE('',*,*,#35249,.F.);
#48877=ORIENTED_EDGE('',*,*,#35234,.T.);
#48878=ORIENTED_EDGE('',*,*,#35231,.T.);
#48879=ORIENTED_EDGE('',*,*,#35219,.T.);
#48880=ORIENTED_EDGE('',*,*,#35214,.T.);
#58972=ADVANCED_FACE('',(#5872),#887,.F.);
#58973=ADVANCED_FACE('',(#5873),#888,.F.);
#58974=ADVANCED_FACE('',(#5874,#1811),#2978,.T.);
#58975=ADVANCED_FACE('',(#5875),#621,.F.);
#58976=ADVANCED_FACE('',(#5876),#889,.F.);
#58977=ADVANCED_FACE('',(#5877),#622,.F.);
#58978=ADVANCED_FACE('',(#5878),#890,.F.);
#58979=ADVANCED_FACE('',(#5879),#891,.F.);
#58980=ADVANCED_FACE('',(#5880),#892,.F.);
#58981=ADVANCED_FACE('',(#5881),#2979,.T.);
#58982=ADVANCED_FACE('',(#5882),#623,.F.);
#58983=ADVANCED_FACE('',(#5883),#893,.F.);
#58984=ADVANCED_FACE('',(#5884),#624,.F.);
#58985=ADVANCED_FACE('',(#5885),#894,.F.);
#58986=ADVANCED_FACE('',(#5886),#625,.F.);
#58987=ADVANCED_FACE('',(#5887),#2980,.T.);
#58988=ADVANCED_FACE('',(#5888),#895,.F.);
#58989=ADVANCED_FACE('',(#5889),#2981,.T.);
#58990=ADVANCED_FACE('',(#5890),#626,.F.);
#58991=ADVANCED_FACE('',(#5891),#896,.F.);
#58992=ADVANCED_FACE('',(#5892,#1812,#1813,#1814,#1815,#1816,#1817),#2982,
 .T.);
#58993=ADVANCED_FACE('',(#5893),#627,.F.);
#58994=ADVANCED_FACE('',(#5894),#897,.F.);
#58995=ADVANCED_FACE('',(#5895),#628,.F.);
#58996=ADVANCED_FACE('',(#5896),#2983,.T.);
#58997=ADVANCED_FACE('',(#5897),#2984,.T.);
#58998=ADVANCED_FACE('',(#5898),#2985,.T.);
#58999=ADVANCED_FACE('',(#5899),#2986,.T.);
#59000=ADVANCED_FACE('',(#5900),#2987,.T.);
#59001=ADVANCED_FACE('',(#5901),#2988,.T.);
#59002=ADVANCED_FACE('',(#5902),#898,.F.);
#59003=ADVANCED_FACE('',(#5903),#629,.F.);
#59004=ADVANCED_FACE('',(#5904),#899,.F.);
#59005=ADVANCED_FACE('',(#5905),#630,.F.);
#59006=ADVANCED_FACE('',(#5906),#900,.F.);
#59007=ADVANCED_FACE('',(#5907),#631,.F.);
#59008=ADVANCED_FACE('',(#5908),#901,.F.);
#59009=ADVANCED_FACE('',(#5909),#632,.F.);
#59010=ADVANCED_FACE('',(#5910),#902,.F.);
#59011=ADVANCED_FACE('',(#5911),#903,.F.);
#59012=ADVANCED_FACE('',(#5912),#904,.F.);
#59013=ADVANCED_FACE('',(#5913),#905,.F.);
#59014=ADVANCED_FACE('',(#5914),#906,.F.);
#59015=ADVANCED_FACE('',(#5915),#633,.F.);
#59016=ADVANCED_FACE('',(#5916),#907,.F.);
#59017=ADVANCED_FACE('',(#5917),#634,.F.);
#59018=ADVANCED_FACE('',(#5918,#1818),#2989,.T.);
#59019=ADVANCED_FACE('',(#5919),#2990,.F.);
#59020=ADVANCED_FACE('',(#5920),#2991,.F.);
#59021=ADVANCED_FACE('',(#5921),#2992,.F.);
#59022=ADVANCED_FACE('',(#5922),#2993,.F.);
#59023=ADVANCED_FACE('',(#5923),#2994,.F.);
#59024=ADVANCED_FACE('',(#5924),#2995,.F.);
#59025=ADVANCED_FACE('',(#5925,#1819,#1820,#1821),#2996,.F.);
#59026=ADVANCED_FACE('',(#5926),#2997,.F.);
#59027=ADVANCED_FACE('',(#5927),#2998,.T.);
#59028=ADVANCED_FACE('',(#5928),#2999,.T.);
#59029=ADVANCED_FACE('',(#5929),#3000,.T.);
#59030=ADVANCED_FACE('',(#5930),#3001,.T.);
#59031=ADVANCED_FACE('',(#5931),#3002,.T.);
#59032=ADVANCED_FACE('',(#5932),#3003,.T.);
#59033=ADVANCED_FACE('',(#5933),#3004,.T.);
#59034=ADVANCED_FACE('',(#5934),#3005,.T.);
#59035=ADVANCED_FACE('',(#5935),#3006,.T.);
#59036=ADVANCED_FACE('',(#5936),#3007,.T.);
#59037=ADVANCED_FACE('',(#5937),#3008,.T.);
#59038=ADVANCED_FACE('',(#5938),#3009,.T.);
#59039=ADVANCED_FACE('',(#5939),#3010,.T.);
#59040=ADVANCED_FACE('',(#5940),#3011,.T.);
#59041=ADVANCED_FACE('',(#5941),#3012,.T.);
#59042=ADVANCED_FACE('',(#5942),#3013,.T.);
#59043=ADVANCED_FACE('',(#5943),#3014,.T.);
#59044=ADVANCED_FACE('',(#5944),#3015,.T.);
#59045=ADVANCED_FACE('',(#5945),#3016,.T.);
#59046=ADVANCED_FACE('',(#5946),#3017,.T.);
#59047=ADVANCED_FACE('',(#5947),#3018,.T.);
#59048=ADVANCED_FACE('',(#5948),#3019,.T.);
#59049=ADVANCED_FACE('',(#5949),#3020,.T.);
#60393=CLOSED_SHELL('',(#58972,#58973,#58974,#58975,#58976,#58977,#58978,
#58979,#58980,#58981,#58982,#58983,#58984,#58985,#58986,#58987,#58988,#58989,
#58990,#58991,#58992,#58993,#58994,#58995,#58996,#58997,#58998,#58999,#59000,
#59001,#59002,#59003,#59004,#59005,#59006,#59007,#59008,#59009,#59010,#59011,
#59012,#59013,#59014,#59015,#59016,#59017,#59018,#59019,#59020,#59021,#59022,
#59023,#59024,#59025,#59026,#59027,#59028,#59029,#59030,#59031,#59032,#59033,
#59034,#59035,#59036,#59037,#59038,#59039,#59040,#59041,#59042,#59043,#59044,
#59045,#59046,#59047,#59048,#59049));
#61812=AXIS2_PLACEMENT_3D('',#92143,#69462,#69463);
#61813=AXIS2_PLACEMENT_3D('',#92144,#69464,#69465);
#61814=AXIS2_PLACEMENT_3D('',#92149,#69467,#69468);
#61815=AXIS2_PLACEMENT_3D('',#92154,#69469,#69470);
#61816=AXIS2_PLACEMENT_3D('',#92155,#69471,#69472);
#61817=AXIS2_PLACEMENT_3D('',#92158,#69473,#69474);
#61818=AXIS2_PLACEMENT_3D('',#92161,#69476,#69477);
#61819=AXIS2_PLACEMENT_3D('',#92162,#69478,#69479);
#61820=AXIS2_PLACEMENT_3D('',#92163,#69480,#69481);
#61821=AXIS2_PLACEMENT_3D('',#92170,#69484,#69485);
#61822=AXIS2_PLACEMENT_3D('',#92171,#69486,#69487);
#61823=AXIS2_PLACEMENT_3D('',#92179,#69492,#69493);
#61824=AXIS2_PLACEMENT_3D('',#92180,#69494,#69495);
#61825=AXIS2_PLACEMENT_3D('',#92183,#69497,#69498);
#61826=AXIS2_PLACEMENT_3D('',#92184,#69499,#69500);
#61827=AXIS2_PLACEMENT_3D('',#92187,#69502,#69503);
#61828=AXIS2_PLACEMENT_3D('',#92188,#69504,#69505);
#61829=AXIS2_PLACEMENT_3D('',#92191,#69507,#69508);
#61830=AXIS2_PLACEMENT_3D('',#92192,#69509,#69510);
#61831=AXIS2_PLACEMENT_3D('',#92195,#69512,#69513);
#61832=AXIS2_PLACEMENT_3D('',#92198,#69515,#69516);
#61833=AXIS2_PLACEMENT_3D('',#92205,#69517,#69518);
#61834=AXIS2_PLACEMENT_3D('',#92208,#69520,#69521);
#61835=AXIS2_PLACEMENT_3D('',#92209,#69522,#69523);
#61836=AXIS2_PLACEMENT_3D('',#92210,#69524,#69525);
#61837=AXIS2_PLACEMENT_3D('',#92231,#69533,#69534);
#61838=AXIS2_PLACEMENT_3D('',#92234,#69536,#69537);
#61839=AXIS2_PLACEMENT_3D('',#92235,#69538,#69539);
#61840=AXIS2_PLACEMENT_3D('',#92237,#69540,#69541);
#61841=AXIS2_PLACEMENT_3D('',#92240,#69543,#69544);
#61842=AXIS2_PLACEMENT_3D('',#92241,#69545,#69546);
#61843=AXIS2_PLACEMENT_3D('',#92242,#69547,#69548);
#61844=AXIS2_PLACEMENT_3D('',#92245,#69550,#69551);
#61845=AXIS2_PLACEMENT_3D('',#92246,#69552,#69553);
#61846=AXIS2_PLACEMENT_3D('',#92247,#69554,#69555);
#61847=AXIS2_PLACEMENT_3D('',#92248,#69556,#69557);
#61848=AXIS2_PLACEMENT_3D('',#92249,#69558,#69559);
#61849=AXIS2_PLACEMENT_3D('',#92252,#69561,#69562);
#61850=AXIS2_PLACEMENT_3D('',#92253,#69563,#69564);
#61851=AXIS2_PLACEMENT_3D('',#92259,#69568,#69569);
#61852=AXIS2_PLACEMENT_3D('',#92266,#69570,#69571);
#61853=AXIS2_PLACEMENT_3D('',#92269,#69573,#69574);
#61854=AXIS2_PLACEMENT_3D('',#92270,#69575,#69576);
#61855=AXIS2_PLACEMENT_3D('',#92271,#69577,#69578);
#61856=AXIS2_PLACEMENT_3D('',#92278,#69583,#69584);
#61857=AXIS2_PLACEMENT_3D('',#92282,#69586,#69587);
#61858=AXIS2_PLACEMENT_3D('',#92284,#69588,#69589);
#61859=AXIS2_PLACEMENT_3D('',#92285,#69590,#69591);
#61860=AXIS2_PLACEMENT_3D('',#92286,#69592,#69593);
#61861=AXIS2_PLACEMENT_3D('',#92288,#69594,#69595);
#61862=AXIS2_PLACEMENT_3D('',#92291,#69597,#69598);
#61863=AXIS2_PLACEMENT_3D('',#92292,#69599,#69600);
#61864=AXIS2_PLACEMENT_3D('',#92299,#69604,#69605);
#61865=AXIS2_PLACEMENT_3D('',#92301,#69606,#69607);
#61866=AXIS2_PLACEMENT_3D('',#92303,#69608,#69609);
#61867=AXIS2_PLACEMENT_3D('',#92305,#69610,#69611);
#61868=AXIS2_PLACEMENT_3D('',#92307,#69612,#69613);
#61869=AXIS2_PLACEMENT_3D('',#92308,#69614,#69615);
#61870=AXIS2_PLACEMENT_3D('',#92312,#69617,#69618);
#61871=AXIS2_PLACEMENT_3D('',#92314,#69619,#69620);
#61872=AXIS2_PLACEMENT_3D('',#92315,#69621,#69622);
#61873=AXIS2_PLACEMENT_3D('',#92316,#69623,#69624);
#61874=AXIS2_PLACEMENT_3D('',#92319,#69626,#69627);
#61875=AXIS2_PLACEMENT_3D('',#92320,#69628,#69629);
#61876=AXIS2_PLACEMENT_3D('',#92324,#69631,#69632);
#61877=AXIS2_PLACEMENT_3D('',#92326,#69633,#69634);
#61878=AXIS2_PLACEMENT_3D('',#92327,#69635,#69636);
#61879=AXIS2_PLACEMENT_3D('',#92328,#69637,#69638);
#61880=AXIS2_PLACEMENT_3D('',#92330,#69640,#69641);
#61881=AXIS2_PLACEMENT_3D('',#92332,#69643,#69644);
#61882=AXIS2_PLACEMENT_3D('',#92334,#69646,#69647);
#61883=AXIS2_PLACEMENT_3D('',#92336,#69649,#69650);
#61884=AXIS2_PLACEMENT_3D('',#92338,#69652,#69653);
#61885=AXIS2_PLACEMENT_3D('',#92340,#69655,#69656);
#61886=AXIS2_PLACEMENT_3D('',#92343,#69658,#69659);
#61887=AXIS2_PLACEMENT_3D('',#92344,#69660,#69661);
#61888=AXIS2_PLACEMENT_3D('',#92347,#69663,#69664);
#61889=AXIS2_PLACEMENT_3D('',#92348,#69665,#69666);
#61890=AXIS2_PLACEMENT_3D('',#92351,#69668,#69669);
#61891=AXIS2_PLACEMENT_3D('',#92352,#69670,#69671);
#61892=AXIS2_PLACEMENT_3D('',#92355,#69673,#69674);
#61893=AXIS2_PLACEMENT_3D('',#92356,#69675,#69676);
#61894=AXIS2_PLACEMENT_3D('',#92359,#69678,#69679);
#61895=AXIS2_PLACEMENT_3D('',#92360,#69680,#69681);
#61896=AXIS2_PLACEMENT_3D('',#92363,#69683,#69684);
#61897=AXIS2_PLACEMENT_3D('',#92364,#69685,#69686);
#61898=AXIS2_PLACEMENT_3D('',#92367,#69688,#69689);
#61899=AXIS2_PLACEMENT_3D('',#92368,#69690,#69691);
#61900=AXIS2_PLACEMENT_3D('',#92371,#69693,#69694);
#61901=AXIS2_PLACEMENT_3D('',#92372,#69695,#69696);
#61902=AXIS2_PLACEMENT_3D('',#92375,#69698,#69699);
#61903=AXIS2_PLACEMENT_3D('',#92378,#69701,#69702);
#61904=AXIS2_PLACEMENT_3D('',#92381,#69704,#69705);
#61905=AXIS2_PLACEMENT_3D('',#92384,#69707,#69708);
#61906=AXIS2_PLACEMENT_3D('',#92388,#69710,#69711);
#61907=AXIS2_PLACEMENT_3D('',#92389,#69712,#69713);
#61908=AXIS2_PLACEMENT_3D('',#92390,#69714,#69715);
#61909=AXIS2_PLACEMENT_3D('',#92397,#69720,#69721);
#61910=AXIS2_PLACEMENT_3D('',#92401,#69723,#69724);
#61911=AXIS2_PLACEMENT_3D('',#92404,#69726,#69727);
#61912=AXIS2_PLACEMENT_3D('',#92405,#69728,#69729);
#61913=AXIS2_PLACEMENT_3D('',#92409,#69731,#69732);
#61914=AXIS2_PLACEMENT_3D('',#92410,#69733,#69734);
#61915=AXIS2_PLACEMENT_3D('',#92412,#69735,#69736);
#61916=AXIS2_PLACEMENT_3D('',#92414,#69738,#69739);
#61917=AXIS2_PLACEMENT_3D('',#92416,#69741,#69742);
#61918=AXIS2_PLACEMENT_3D('',#92426,#69748,#69749);
#61919=AXIS2_PLACEMENT_3D('',#92432,#69753,#69754);
#61920=AXIS2_PLACEMENT_3D('',#92438,#69758,#69759);
#61921=AXIS2_PLACEMENT_3D('',#92456,#69769,#69770);
#61922=AXIS2_PLACEMENT_3D('',#92460,#69773,#69774);
#61923=AXIS2_PLACEMENT_3D('',#92468,#69779,#69780);
#61924=AXIS2_PLACEMENT_3D('',#92478,#69786,#69787);
#61925=AXIS2_PLACEMENT_3D('',#92480,#69789,#69790);
#61926=AXIS2_PLACEMENT_3D('',#92484,#69793,#69794);
#61927=AXIS2_PLACEMENT_3D('',#92487,#69797,#69798);
#61928=AXIS2_PLACEMENT_3D('',#92491,#69801,#69802);
#61929=AXIS2_PLACEMENT_3D('',#92495,#69805,#69806);
#61930=AXIS2_PLACEMENT_3D('',#92498,#69809,#69810);
#61931=AXIS2_PLACEMENT_3D('',#92502,#69813,#69814);
#61932=AXIS2_PLACEMENT_3D('',#92505,#69817,#69818);
#61933=AXIS2_PLACEMENT_3D('',#92509,#69821,#69822);
#61934=AXIS2_PLACEMENT_3D('',#92512,#69825,#69826);
#61935=AXIS2_PLACEMENT_3D('',#92517,#69830,#69831);
#61936=AXIS2_PLACEMENT_3D('',#92519,#69833,#69834);
#61937=AXIS2_PLACEMENT_3D('',#92523,#69838,#69839);
#61938=AXIS2_PLACEMENT_3D('',#92524,#69840,#69841);
#61939=AXIS2_PLACEMENT_3D('',#92525,#69842,#69843);
#61940=AXIS2_PLACEMENT_3D('',#92526,#69844,#69845);
#61941=AXIS2_PLACEMENT_3D('',#92528,#69847,#69848);
#61942=AXIS2_PLACEMENT_3D('',#92530,#69850,#69851);
#61943=AXIS2_PLACEMENT_3D('',#92531,#69852,#69853);
#61944=AXIS2_PLACEMENT_3D('',#92534,#69856,#69857);
#61945=AXIS2_PLACEMENT_3D('',#92535,#69858,#69859);
#61946=AXIS2_PLACEMENT_3D('',#92537,#69861,#69862);
#61947=AXIS2_PLACEMENT_3D('',#92538,#69863,#69864);
#69462=DIRECTION('axis',(0.,0.,1.));
#69463=DIRECTION('refdir',(1.,0.,0.));
#69464=DIRECTION('center_axis',(0.,0.,-1.));
#69465=DIRECTION('ref_axis',(1.,0.,0.));
#69466=DIRECTION('',(0.707106781186548,-8.65956056235494E-17,0.707106781186548));
#69467=DIRECTION('center_axis',(0.,0.,-1.));
#69468=DIRECTION('ref_axis',(1.,0.,0.));
#69469=DIRECTION('center_axis',(0.,0.,1.));
#69470=DIRECTION('ref_axis',(1.,0.,0.));
#69471=DIRECTION('center_axis',(0.,0.,1.));
#69472=DIRECTION('ref_axis',(1.,0.,0.));
#69473=DIRECTION('center_axis',(0.,0.,1.));
#69474=DIRECTION('ref_axis',(1.,0.,0.));
#69475=DIRECTION('',(0.707106781186568,8.65956056235519E-17,-0.707106781186527));
#69476=DIRECTION('center_axis',(0.,0.,-1.));
#69477=DIRECTION('ref_axis',(1.,0.,0.));
#69478=DIRECTION('center_axis',(0.,0.,1.));
#69479=DIRECTION('ref_axis',(1.,0.,0.));
#69480=DIRECTION('center_axis',(0.,0.,1.));
#69481=DIRECTION('ref_axis',(0.,-1.,0.));
#69482=DIRECTION('',(0.,1.,0.));
#69483=DIRECTION('',(-1.,0.,0.));
#69484=DIRECTION('center_axis',(0.,0.,1.));
#69485=DIRECTION('ref_axis',(1.,0.,0.));
#69486=DIRECTION('center_axis',(0.,0.,1.));
#69487=DIRECTION('ref_axis',(1.,0.,0.));
#69488=DIRECTION('',(-1.,0.,0.));
#69489=DIRECTION('',(-1.,0.,0.));
#69490=DIRECTION('',(0.,-1.,0.));
#69491=DIRECTION('',(1.,0.,0.));
#69492=DIRECTION('center_axis',(0.,0.,1.));
#69493=DIRECTION('ref_axis',(1.,0.,0.));
#69494=DIRECTION('center_axis',(0.,0.,-1.));
#69495=DIRECTION('ref_axis',(1.,0.,0.));
#69496=DIRECTION('',(0.,0.,-1.));
#69497=DIRECTION('center_axis',(0.,0.,-1.));
#69498=DIRECTION('ref_axis',(1.,0.,0.));
#69499=DIRECTION('center_axis',(0.,0.,1.));
#69500=DIRECTION('ref_axis',(1.,0.,0.));
#69501=DIRECTION('',(0.707106781186568,8.65956056235519E-17,-0.707106781186527));
#69502=DIRECTION('center_axis',(0.,0.,-1.));
#69503=DIRECTION('ref_axis',(1.,0.,0.));
#69504=DIRECTION('center_axis',(0.,0.,-1.));
#69505=DIRECTION('ref_axis',(1.,0.,0.));
#69506=DIRECTION('',(0.,0.,-1.));
#69507=DIRECTION('center_axis',(0.,0.,-1.));
#69508=DIRECTION('ref_axis',(1.,0.,0.));
#69509=DIRECTION('center_axis',(0.,0.,1.));
#69510=DIRECTION('ref_axis',(1.,0.,0.));
#69511=DIRECTION('',(-0.857167300702113,-1.04972719113862E-16,0.515038074910054));
#69512=DIRECTION('center_axis',(0.,0.,1.));
#69513=DIRECTION('ref_axis',(1.,0.,0.));
#69514=DIRECTION('',(-0.857167300702109,-1.04972719113861E-16,0.51503807491006));
#69515=DIRECTION('center_axis',(0.,0.,-1.));
#69516=DIRECTION('ref_axis',(1.,0.,0.));
#69517=DIRECTION('center_axis',(0.,0.,-1.));
#69518=DIRECTION('ref_axis',(1.,0.,0.));
#69519=DIRECTION('',(0.707106781186552,-8.65956056235499E-17,0.707106781186543));
#69520=DIRECTION('center_axis',(0.,0.,1.));
#69521=DIRECTION('ref_axis',(1.,0.,0.));
#69522=DIRECTION('center_axis',(0.,0.,-1.));
#69523=DIRECTION('ref_axis',(1.,0.,0.));
#69524=DIRECTION('center_axis',(0.,-0.707106781186546,-0.707106781186549));
#69525=DIRECTION('ref_axis',(-1.,0.,0.));
#69526=DIRECTION('',(1.,0.,0.));
#69527=DIRECTION('',(0.,-0.707106781186549,0.707106781186546));
#69528=DIRECTION('',(-1.,0.,0.));
#69529=DIRECTION('',(0.,0.707106781186549,-0.707106781186546));
#69530=DIRECTION('',(1.,0.,0.));
#69531=DIRECTION('',(1.,0.,0.));
#69532=DIRECTION('',(1.,0.,0.));
#69533=DIRECTION('center_axis',(0.,0.,1.));
#69534=DIRECTION('ref_axis',(1.,0.,0.));
#69535=DIRECTION('',(0.,0.,1.));
#69536=DIRECTION('center_axis',(0.,-0.5,-0.866025403784439));
#69537=DIRECTION('ref_axis',(0.,0.866025403784439,-0.5));
#69538=DIRECTION('center_axis',(0.,0.,-1.));
#69539=DIRECTION('ref_axis',(1.,0.,0.));
#69540=DIRECTION('center_axis',(0.,0.,-1.));
#69541=DIRECTION('ref_axis',(1.,0.,0.));
#69542=DIRECTION('',(0.707106781186552,-8.65956056235499E-17,0.707106781186543));
#69543=DIRECTION('center_axis',(0.,0.,1.));
#69544=DIRECTION('ref_axis',(1.,0.,0.));
#69545=DIRECTION('center_axis',(0.,0.,-1.));
#69546=DIRECTION('ref_axis',(1.,0.,0.));
#69547=DIRECTION('center_axis',(0.,0.,1.));
#69548=DIRECTION('ref_axis',(1.,0.,0.));
#69549=DIRECTION('',(0.,0.,1.));
#69550=DIRECTION('center_axis',(0.,-0.5,-0.866025403784439));
#69551=DIRECTION('ref_axis',(0.,0.866025403784439,-0.5));
#69552=DIRECTION('center_axis',(0.,0.,-1.));
#69553=DIRECTION('ref_axis',(1.,0.,0.));
#69554=DIRECTION('center_axis',(0.,0.,1.));
#69555=DIRECTION('ref_axis',(1.,0.,0.));
#69556=DIRECTION('center_axis',(0.,0.,-1.));
#69557=DIRECTION('ref_axis',(1.,0.,0.));
#69558=DIRECTION('center_axis',(0.,0.,1.));
#69559=DIRECTION('ref_axis',(1.,0.,0.));
#69560=DIRECTION('',(0.,0.,1.));
#69561=DIRECTION('center_axis',(0.,-0.5,-0.866025403784439));
#69562=DIRECTION('ref_axis',(0.,0.866025403784439,-0.5));
#69563=DIRECTION('center_axis',(0.,0.,-1.));
#69564=DIRECTION('ref_axis',(0.,1.,0.));
#69565=DIRECTION('',(0.,-1.,0.));
#69566=DIRECTION('',(-1.,0.,0.));
#69567=DIRECTION('',(0.,1.,0.));
#69568=DIRECTION('center_axis',(0.,1.,0.));
#69569=DIRECTION('ref_axis',(1.,0.,0.));
#69570=DIRECTION('center_axis',(0.,1.,0.));
#69571=DIRECTION('ref_axis',(1.,0.,0.));
#69572=DIRECTION('',(0.707106781186537,-0.707106781186558,-8.6595605623548E-17));
#69573=DIRECTION('center_axis',(0.,-1.,0.));
#69574=DIRECTION('ref_axis',(1.,0.,0.));
#69575=DIRECTION('center_axis',(0.,1.,0.));
#69576=DIRECTION('ref_axis',(1.,0.,0.));
#69577=DIRECTION('center_axis',(0.,0.707106781186548,0.707106781186548));
#69578=DIRECTION('ref_axis',(1.,0.,0.));
#69579=DIRECTION('',(-1.,0.,0.));
#69580=DIRECTION('',(0.,-0.707106781186548,0.707106781186548));
#69581=DIRECTION('',(0.,0.707106781186548,-0.707106781186548));
#69582=DIRECTION('',(-1.,0.,0.));
#69583=DIRECTION('center_axis',(0.,-1.,0.));
#69584=DIRECTION('ref_axis',(1.,0.,0.));
#69585=DIRECTION('',(0.,-1.,0.));
#69586=DIRECTION('center_axis',(0.,-1.,0.));
#69587=DIRECTION('ref_axis',(1.,0.,0.));
#69588=DIRECTION('center_axis',(0.,-1.,0.));
#69589=DIRECTION('ref_axis',(1.,0.,0.));
#69590=DIRECTION('center_axis',(0.,-1.,0.));
#69591=DIRECTION('ref_axis',(1.,0.,0.));
#69592=DIRECTION('center_axis',(0.,1.,0.));
#69593=DIRECTION('ref_axis',(1.,0.,0.));
#69594=DIRECTION('center_axis',(0.,1.,0.));
#69595=DIRECTION('ref_axis',(1.,0.,0.));
#69596=DIRECTION('',(0.707106781186558,-0.707106781186537,-8.65956056235506E-17));
#69597=DIRECTION('center_axis',(0.,-1.,0.));
#69598=DIRECTION('ref_axis',(1.,0.,0.));
#69599=DIRECTION('center_axis',(0.,1.,0.));
#69600=DIRECTION('ref_axis',(0.,0.,1.));
#69601=DIRECTION('',(0.,0.,1.));
#69602=DIRECTION('',(1.,0.,0.));
#69603=DIRECTION('',(0.,0.,-1.));
#69604=DIRECTION('center_axis',(0.,1.,0.));
#69605=DIRECTION('ref_axis',(1.,0.,0.));
#69606=DIRECTION('center_axis',(0.,1.,0.));
#69607=DIRECTION('ref_axis',(1.,0.,0.));
#69608=DIRECTION('center_axis',(0.,1.,0.));
#69609=DIRECTION('ref_axis',(1.,0.,0.));
#69610=DIRECTION('center_axis',(0.,1.,0.));
#69611=DIRECTION('ref_axis',(1.,0.,0.));
#69612=DIRECTION('center_axis',(0.,1.,0.));
#69613=DIRECTION('ref_axis',(1.,0.,0.));
#69614=DIRECTION('center_axis',(0.,-1.,0.));
#69615=DIRECTION('ref_axis',(1.,0.,0.));
#69616=DIRECTION('',(0.,-1.,0.));
#69617=DIRECTION('center_axis',(0.,-1.,0.));
#69618=DIRECTION('ref_axis',(1.,0.,0.));
#69619=DIRECTION('center_axis',(0.,-1.,0.));
#69620=DIRECTION('ref_axis',(1.,0.,0.));
#69621=DIRECTION('center_axis',(0.,-1.,0.));
#69622=DIRECTION('ref_axis',(1.,0.,0.));
#69623=DIRECTION('center_axis',(0.,1.,0.));
#69624=DIRECTION('ref_axis',(1.,0.,0.));
#69625=DIRECTION('',(0.707106781186558,-0.707106781186537,-8.65956056235506E-17));
#69626=DIRECTION('center_axis',(0.,-1.,0.));
#69627=DIRECTION('ref_axis',(1.,0.,0.));
#69628=DIRECTION('center_axis',(0.,-1.,0.));
#69629=DIRECTION('ref_axis',(1.,0.,0.));
#69630=DIRECTION('',(0.,-1.,0.));
#69631=DIRECTION('center_axis',(0.,-1.,0.));
#69632=DIRECTION('ref_axis',(1.,0.,0.));
#69633=DIRECTION('center_axis',(0.,-1.,0.));
#69634=DIRECTION('ref_axis',(1.,0.,0.));
#69635=DIRECTION('center_axis',(0.,-1.,0.));
#69636=DIRECTION('ref_axis',(1.,0.,0.));
#69637=DIRECTION('center_axis',(0.,1.,0.));
#69638=DIRECTION('ref_axis',(1.,0.,0.));
#69639=DIRECTION('',(0.,0.,1.));
#69640=DIRECTION('center_axis',(0.,1.,0.));
#69641=DIRECTION('ref_axis',(1.,0.,0.));
#69642=DIRECTION('',(0.,0.,1.));
#69643=DIRECTION('center_axis',(0.,1.,0.));
#69644=DIRECTION('ref_axis',(1.,0.,0.));
#69645=DIRECTION('',(0.,0.,1.));
#69646=DIRECTION('center_axis',(0.,1.,0.));
#69647=DIRECTION('ref_axis',(1.,0.,0.));
#69648=DIRECTION('',(0.,0.,1.));
#69649=DIRECTION('center_axis',(0.,1.,0.));
#69650=DIRECTION('ref_axis',(1.,0.,0.));
#69651=DIRECTION('',(0.,0.,1.));
#69652=DIRECTION('center_axis',(0.,1.,0.));
#69653=DIRECTION('ref_axis',(1.,0.,0.));
#69654=DIRECTION('',(0.,0.,1.));
#69655=DIRECTION('center_axis',(0.,1.,0.));
#69656=DIRECTION('ref_axis',(1.,0.,0.));
#69657=DIRECTION('',(0.707106781186554,-0.707106781186541,-8.65956056235501E-17));
#69658=DIRECTION('center_axis',(0.,-1.,0.));
#69659=DIRECTION('ref_axis',(1.,0.,0.));
#69660=DIRECTION('center_axis',(0.,-1.,0.));
#69661=DIRECTION('ref_axis',(1.,0.,0.));
#69662=DIRECTION('',(0.,-1.,0.));
#69663=DIRECTION('center_axis',(0.,-1.,0.));
#69664=DIRECTION('ref_axis',(1.,0.,0.));
#69665=DIRECTION('center_axis',(0.,1.,0.));
#69666=DIRECTION('ref_axis',(1.,0.,0.));
#69667=DIRECTION('',(0.707106781186554,-0.707106781186541,-8.65956056235501E-17));
#69668=DIRECTION('center_axis',(0.,-1.,0.));
#69669=DIRECTION('ref_axis',(1.,0.,0.));
#69670=DIRECTION('center_axis',(0.,-1.,0.));
#69671=DIRECTION('ref_axis',(1.,0.,0.));
#69672=DIRECTION('',(0.,-1.,0.));
#69673=DIRECTION('center_axis',(0.,-1.,0.));
#69674=DIRECTION('ref_axis',(1.,0.,0.));
#69675=DIRECTION('center_axis',(0.,1.,0.));
#69676=DIRECTION('ref_axis',(1.,0.,0.));
#69677=DIRECTION('',(0.707106781186554,-0.707106781186541,-8.65956056235501E-17));
#69678=DIRECTION('center_axis',(0.,-1.,0.));
#69679=DIRECTION('ref_axis',(1.,0.,0.));
#69680=DIRECTION('center_axis',(0.,-1.,0.));
#69681=DIRECTION('ref_axis',(1.,0.,0.));
#69682=DIRECTION('',(0.,-1.,0.));
#69683=DIRECTION('center_axis',(0.,-1.,0.));
#69684=DIRECTION('ref_axis',(1.,0.,0.));
#69685=DIRECTION('center_axis',(0.,1.,0.));
#69686=DIRECTION('ref_axis',(1.,0.,0.));
#69687=DIRECTION('',(0.707106781186554,-0.707106781186541,-8.65956056235501E-17));
#69688=DIRECTION('center_axis',(0.,-1.,0.));
#69689=DIRECTION('ref_axis',(1.,0.,0.));
#69690=DIRECTION('center_axis',(0.,-1.,0.));
#69691=DIRECTION('ref_axis',(1.,0.,0.));
#69692=DIRECTION('',(0.,-1.,0.));
#69693=DIRECTION('center_axis',(0.,-1.,0.));
#69694=DIRECTION('ref_axis',(1.,0.,0.));
#69695=DIRECTION('center_axis',(0.,1.,0.));
#69696=DIRECTION('ref_axis',(1.,0.,0.));
#69697=DIRECTION('',(0.857167300702111,-0.515038074910056,1.04972719113862E-16));
#69698=DIRECTION('center_axis',(0.,1.,0.));
#69699=DIRECTION('ref_axis',(1.,0.,0.));
#69700=DIRECTION('',(0.857167300702111,-0.515038074910056,1.04972719113862E-16));
#69701=DIRECTION('center_axis',(0.,1.,0.));
#69702=DIRECTION('ref_axis',(1.,0.,0.));
#69703=DIRECTION('',(0.857167300702111,-0.515038074910056,1.04972719113862E-16));
#69704=DIRECTION('center_axis',(0.,1.,0.));
#69705=DIRECTION('ref_axis',(1.,0.,0.));
#69706=DIRECTION('',(0.857167300702111,-0.515038074910056,1.04972719113862E-16));
#69707=DIRECTION('center_axis',(0.,0.,1.));
#69708=DIRECTION('ref_axis',(1.,0.,0.));
#69709=DIRECTION('',(0.707106781186537,8.6595605623548E-17,-0.707106781186558));
#69710=DIRECTION('center_axis',(0.,0.,-1.));
#69711=DIRECTION('ref_axis',(1.,0.,0.));
#69712=DIRECTION('center_axis',(0.,0.,-1.));
#69713=DIRECTION('ref_axis',(1.,0.,0.));
#69714=DIRECTION('center_axis',(0.,0.,-1.));
#69715=DIRECTION('ref_axis',(6.12323399573677E-17,-1.,0.));
#69716=DIRECTION('',(0.,0.,-1.));
#69717=DIRECTION('',(0.,0.,-1.));
#69718=DIRECTION('',(0.,0.,-1.));
#69719=DIRECTION('',(0.,0.,-1.));
#69720=DIRECTION('center_axis',(0.,0.,-1.));
#69721=DIRECTION('ref_axis',(1.,0.,0.));
#69722=DIRECTION('',(0.,0.,-1.));
#69723=DIRECTION('center_axis',(0.,0.,1.));
#69724=DIRECTION('ref_axis',(1.,0.,0.));
#69725=DIRECTION('',(0.,0.,1.));
#69726=DIRECTION('center_axis',(0.,0.,-1.));
#69727=DIRECTION('ref_axis',(1.,0.,0.));
#69728=DIRECTION('center_axis',(0.,0.,1.));
#69729=DIRECTION('ref_axis',(1.,0.,0.));
#69730=DIRECTION('',(-0.857167300702114,-1.04972719113862E-16,0.515038074910052));
#69731=DIRECTION('center_axis',(0.,0.,-1.));
#69732=DIRECTION('ref_axis',(1.,0.,0.));
#69733=DIRECTION('center_axis',(0.,0.,-1.));
#69734=DIRECTION('ref_axis',(1.,0.,0.));
#69735=DIRECTION('center_axis',(0.,0.,-1.));
#69736=DIRECTION('ref_axis',(1.,0.,0.));
#69737=DIRECTION('',(0.,0.,-1.));
#69738=DIRECTION('center_axis',(0.,0.,1.));
#69739=DIRECTION('ref_axis',(1.,0.,0.));
#69740=DIRECTION('',(-1.,0.,0.));
#69741=DIRECTION('center_axis',(0.,1.,0.));
#69742=DIRECTION('ref_axis',(0.,0.,1.));
#69743=DIRECTION('',(1.,0.,0.));
#69744=DIRECTION('',(0.,0.,1.));
#69745=DIRECTION('',(1.,0.,0.));
#69746=DIRECTION('',(0.,0.,-1.));
#69747=DIRECTION('',(1.,0.,0.));
#69748=DIRECTION('center_axis',(0.,0.,-1.));
#69749=DIRECTION('ref_axis',(0.,1.,0.));
#69750=DIRECTION('',(-1.,0.,0.));
#69751=DIRECTION('',(0.,-1.,0.));
#69752=DIRECTION('',(0.,1.,0.));
#69753=DIRECTION('center_axis',(0.,0.,1.));
#69754=DIRECTION('ref_axis',(0.,-1.,0.));
#69755=DIRECTION('',(0.,1.,0.));
#69756=DIRECTION('',(1.,0.,0.));
#69757=DIRECTION('',(0.,-1.,0.));
#69758=DIRECTION('center_axis',(1.,0.,0.));
#69759=DIRECTION('ref_axis',(0.,0.,-1.));
#69760=DIRECTION('',(0.,0.,1.));
#69761=DIRECTION('',(0.,-0.866025403784439,-0.499999999999999));
#69762=DIRECTION('',(0.,0.,-1.));
#69763=DIRECTION('',(0.,-1.,0.));
#69764=DIRECTION('',(0.,0.,1.));
#69765=DIRECTION('',(0.,1.,0.));
#69766=DIRECTION('',(0.,0.,-1.));
#69767=DIRECTION('',(0.,0.866025403784439,-0.5));
#69768=DIRECTION('',(0.,0.,1.));
#69769=DIRECTION('center_axis',(0.,1.,0.));
#69770=DIRECTION('ref_axis',(0.,0.,1.));
#69771=DIRECTION('',(0.,0.,-1.));
#69772=DIRECTION('',(1.,0.,0.));
#69773=DIRECTION('center_axis',(0.,-0.499999999999999,0.866025403784439));
#69774=DIRECTION('ref_axis',(0.,-0.866025403784439,-0.499999999999999));
#69775=DIRECTION('',(0.654653670707982,-0.654653670707974,-0.377964473009224));
#69776=DIRECTION('',(0.,0.866025403784439,0.499999999999999));
#69777=DIRECTION('',(0.654653670707982,0.654653670707974,0.377964473009224));
#69778=DIRECTION('',(1.,0.,0.));
#69779=DIRECTION('center_axis',(0.,-0.5,-0.866025403784439));
#69780=DIRECTION('ref_axis',(0.,0.866025403784439,-0.5));
#69781=DIRECTION('',(-0.654653670707982,0.654653670707974,-0.377964473009225));
#69782=DIRECTION('',(-1.,0.,0.));
#69783=DIRECTION('',(-0.654653670707982,-0.654653670707974,0.377964473009225));
#69784=DIRECTION('',(0.,-0.866025403784439,0.5));
#69785=DIRECTION('',(1.,0.,0.));
#69786=DIRECTION('center_axis',(0.,1.,0.));
#69787=DIRECTION('ref_axis',(0.,0.,1.));
#69788=DIRECTION('',(0.,0.,-1.));
#69789=DIRECTION('center_axis',(-0.707106781186543,-0.707106781186552,0.));
#69790=DIRECTION('ref_axis',(0.,0.,1.));
#69791=DIRECTION('',(0.,0.,1.));
#69792=DIRECTION('',(-0.707106781186552,0.707106781186543,1.25607396694701E-14));
#69793=DIRECTION('center_axis',(-0.707106781186543,-0.707106781186552,0.));
#69794=DIRECTION('ref_axis',(0.,0.,1.));
#69795=DIRECTION('',(0.707106781186552,-0.707106781186543,0.));
#69796=DIRECTION('',(0.,0.,1.));
#69797=DIRECTION('center_axis',(0.,-1.,0.));
#69798=DIRECTION('ref_axis',(0.,0.,-1.));
#69799=DIRECTION('',(0.,0.,-1.));
#69800=DIRECTION('',(1.,0.,0.));
#69801=DIRECTION('center_axis',(0.707106781186543,-0.707106781186552,0.));
#69802=DIRECTION('ref_axis',(0.,0.,-1.));
#69803=DIRECTION('',(0.,0.,1.));
#69804=DIRECTION('',(-0.707106781186552,-0.707106781186543,-1.25607396694701E-14));
#69805=DIRECTION('center_axis',(0.577350269189616,-0.577350269189634,0.577350269189627));
#69806=DIRECTION('ref_axis',(0.707106781186554,0.,-0.707106781186541));
#69807=DIRECTION('',(0.707106781186554,0.,-0.707106781186541));
#69808=DIRECTION('',(0.,0.707106781186543,0.707106781186552));
#69809=DIRECTION('center_axis',(0.577350269189619,0.577350269189629,0.577350269189629));
#69810=DIRECTION('ref_axis',(0.707106781186554,0.,-0.707106781186541));
#69811=DIRECTION('',(0.707106781186554,-0.707106781186541,0.));
#69812=DIRECTION('',(-0.707106781186554,0.,0.707106781186541));
#69813=DIRECTION('center_axis',(-0.577350269189616,-0.577350269189634,0.577350269189627));
#69814=DIRECTION('ref_axis',(0.707106781186554,0.,0.707106781186541));
#69815=DIRECTION('',(0.,-0.707106781186543,-0.707106781186552));
#69816=DIRECTION('',(0.707106781186554,0.,0.707106781186541));
#69817=DIRECTION('center_axis',(0.577350269189621,-0.577350269189627,-0.57735026918963));
#69818=DIRECTION('ref_axis',(-0.707106781186553,0.,-0.707106781186542));
#69819=DIRECTION('',(0.707106781186552,0.707106781186543,0.));
#69820=DIRECTION('',(-0.707106781186552,1.57009245868376E-15,-0.707106781186543));
#69821=DIRECTION('center_axis',(-0.577350269189619,0.577350269189629,0.577350269189629));
#69822=DIRECTION('ref_axis',(0.707106781186554,0.,0.707106781186541));
#69823=DIRECTION('',(0.707106781186554,0.707106781186541,0.));
#69824=DIRECTION('',(-0.707106781186554,0.,-0.707106781186541));
#69825=DIRECTION('center_axis',(0.57735026918962,0.577350269189629,-0.577350269189628));
#69826=DIRECTION('ref_axis',(-0.707106781186552,0.,-0.707106781186543));
#69827=DIRECTION('',(0.707106781186552,0.,0.707106781186543));
#69828=DIRECTION('',(0.,-0.707106781186547,-0.707106781186548));
#69829=DIRECTION('',(-0.707106781186554,0.707106781186541,-1.57009245868377E-15));
#69830=DIRECTION('center_axis',(-0.57735026918962,-0.577350269189628,-0.577350269189629));
#69831=DIRECTION('ref_axis',(-0.707106781186553,0.,0.707106781186542));
#69832=DIRECTION('',(-0.707106781186552,-1.57009245868376E-15,0.707106781186543));
#69833=DIRECTION('center_axis',(-0.57735026918962,0.577350269189629,-0.577350269189628));
#69834=DIRECTION('ref_axis',(-0.707106781186552,0.,0.707106781186543));
#69835=DIRECTION('',(0.707106781186552,0.,-0.707106781186543));
#69836=DIRECTION('',(-0.707106781186554,-0.707106781186541,1.57009245868377E-15));
#69837=DIRECTION('',(0.,0.707106781186547,0.707106781186548));
#69838=DIRECTION('center_axis',(-0.707106781186541,0.707106781186554,0.));
#69839=DIRECTION('ref_axis',(0.,0.,1.));
#69840=DIRECTION('center_axis',(0.,0.707106781186548,-0.707106781186547));
#69841=DIRECTION('ref_axis',(-1.,0.,0.));
#69842=DIRECTION('center_axis',(-0.707106781186543,0.,-0.707106781186552));
#69843=DIRECTION('ref_axis',(-0.707106781186552,0.,0.707106781186543));
#69844=DIRECTION('center_axis',(0.707106781186541,0.707106781186554,0.));
#69845=DIRECTION('ref_axis',(0.,0.,-1.));
#69846=DIRECTION('',(0.,0.,-1.));
#69847=DIRECTION('center_axis',(0.707106781186543,0.,-0.707106781186552));
#69848=DIRECTION('ref_axis',(-0.707106781186552,0.,-0.707106781186543));
#69849=DIRECTION('',(0.,-1.,0.));
#69850=DIRECTION('center_axis',(-0.707106781186541,0.,0.707106781186554));
#69851=DIRECTION('ref_axis',(0.707106781186554,0.,0.707106781186541));
#69852=DIRECTION('center_axis',(0.707106781186543,-0.707106781186552,0.));
#69853=DIRECTION('ref_axis',(0.,0.,-1.));
#69854=DIRECTION('',(0.,0.,-1.));
#69855=DIRECTION('',(0.,0.,1.));
#69856=DIRECTION('center_axis',(0.,-0.707106781186552,0.707106781186543));
#69857=DIRECTION('ref_axis',(1.,0.,0.));
#69858=DIRECTION('center_axis',(0.707106781186541,0.,0.707106781186554));
#69859=DIRECTION('ref_axis',(0.707106781186554,0.,-0.707106781186541));
#69860=DIRECTION('',(0.,1.,0.));
#69861=DIRECTION('center_axis',(0.,-1.,0.));
#69862=DIRECTION('ref_axis',(0.,0.,-1.));
#69863=DIRECTION('center_axis',(1.,0.,0.));
#69864=DIRECTION('ref_axis',(0.,0.,-1.));
#92143=CARTESIAN_POINT('',(0.,0.,0.));
#92144=CARTESIAN_POINT('Origin',(110.,10.75,8.65));
#92145=CARTESIAN_POINT('',(107.65,10.75,8.5));
#92146=CARTESIAN_POINT('',(107.95,10.75,8.8));
#92147=CARTESIAN_POINT('',(107.8,10.75,8.65));
#92148=CARTESIAN_POINT('',(111.568438714136,9.,8.5));
#92149=CARTESIAN_POINT('Origin',(110.,10.75,8.5));
#92150=CARTESIAN_POINT('',(110.,8.7,8.8));
#92151=CARTESIAN_POINT('Ctrl Pts',(111.568438714136,9.,8.5));
#92152=CARTESIAN_POINT('Ctrl Pts',(110.784219357068,8.7,8.8));
#92153=CARTESIAN_POINT('Ctrl Pts',(110.,8.7,8.8));
#92154=CARTESIAN_POINT('Origin',(110.,10.75,8.8));
#92155=CARTESIAN_POINT('Origin',(118.5,10.2,48.425));
#92156=CARTESIAN_POINT('',(118.5,9.,48.5));
#92157=CARTESIAN_POINT('',(117.3,10.2,48.5));
#92158=CARTESIAN_POINT('Origin',(118.5,10.2,48.5));
#92159=CARTESIAN_POINT('',(117.45,10.2,48.35));
#92160=CARTESIAN_POINT('',(117.375,10.2,48.425));
#92161=CARTESIAN_POINT('Origin',(118.5,10.2,48.35));
#92162=CARTESIAN_POINT('Origin',(118.5,10.2,48.5));
#92163=CARTESIAN_POINT('Origin',(90.,28.,48.5));
#92164=CARTESIAN_POINT('',(90.5,9.,48.5));
#92165=CARTESIAN_POINT('',(90.5,27.5,48.5));
#92166=CARTESIAN_POINT('',(90.5,23.125,48.5));
#92167=CARTESIAN_POINT('',(101.5,9.,48.5));
#92168=CARTESIAN_POINT('',(90.,9.,48.5));
#92169=CARTESIAN_POINT('',(100.3,10.2,48.5));
#92170=CARTESIAN_POINT('Origin',(101.5,10.2,48.5));
#92171=CARTESIAN_POINT('Origin',(101.5,10.2,48.5));
#92172=CARTESIAN_POINT('',(90.,9.,48.5));
#92173=CARTESIAN_POINT('',(129.5,9.,48.5));
#92174=CARTESIAN_POINT('',(90.,9.,48.5));
#92175=CARTESIAN_POINT('',(129.5,27.5,48.5));
#92176=CARTESIAN_POINT('',(129.5,23.125,48.5));
#92177=CARTESIAN_POINT('',(90.,27.5,48.5));
#92178=CARTESIAN_POINT('',(104.9,18.,48.5));
#92179=CARTESIAN_POINT('Origin',(110.,18.,48.5));
#92180=CARTESIAN_POINT('Origin',(118.5,10.2,48.5));
#92181=CARTESIAN_POINT('',(117.45,10.2,44.5));
#92182=CARTESIAN_POINT('',(117.45,10.2,48.5));
#92183=CARTESIAN_POINT('Origin',(118.5,10.2,44.5));
#92184=CARTESIAN_POINT('Origin',(101.5,10.2,48.425));
#92185=CARTESIAN_POINT('',(100.45,10.2,48.35));
#92186=CARTESIAN_POINT('',(100.375,10.2,48.425));
#92187=CARTESIAN_POINT('Origin',(101.5,10.2,48.35));
#92188=CARTESIAN_POINT('Origin',(101.5,10.2,48.5));
#92189=CARTESIAN_POINT('',(100.45,10.2,44.5));
#92190=CARTESIAN_POINT('',(100.45,10.2,48.5));
#92191=CARTESIAN_POINT('Origin',(101.5,10.2,44.5));
#92192=CARTESIAN_POINT('Origin',(118.5,10.2,44.1845481750105));
#92193=CARTESIAN_POINT('',(118.5,10.2,43.8690963500211));
#92194=CARTESIAN_POINT('',(117.975,10.2,44.1845481750105));
#92195=CARTESIAN_POINT('Origin',(101.5,10.2,44.1845481750105));
#92196=CARTESIAN_POINT('',(101.5,10.2,43.8690963500211));
#92197=CARTESIAN_POINT('',(100.975,10.2,44.1845481750105));
#92198=CARTESIAN_POINT('Origin',(122.,10.75,8.625));
#92199=CARTESIAN_POINT('',(122.421307488659,9.,8.5));
#92200=CARTESIAN_POINT('',(121.578692511341,9.,8.5));
#92201=CARTESIAN_POINT('Ctrl Pts',(122.421307488659,9.,8.5));
#92202=CARTESIAN_POINT('Ctrl Pts',(122.,8.95,8.55));
#92203=CARTESIAN_POINT('Ctrl Pts',(121.578692511341,9.,8.5));
#92204=CARTESIAN_POINT('',(120.2,10.75,8.5));
#92205=CARTESIAN_POINT('Origin',(122.,10.75,8.5));
#92206=CARTESIAN_POINT('',(120.45,10.75,8.75));
#92207=CARTESIAN_POINT('',(120.325,10.75,8.625));
#92208=CARTESIAN_POINT('Origin',(122.,10.75,8.75));
#92209=CARTESIAN_POINT('Origin',(122.,10.75,8.5));
#92210=CARTESIAN_POINT('Origin',(90.,8.75,8.75));
#92211=CARTESIAN_POINT('',(129.5,9.,8.5));
#92212=CARTESIAN_POINT('',(90.,9.,8.5));
#92213=CARTESIAN_POINT('',(129.5,8.5,9.));
#92214=CARTESIAN_POINT('',(129.5,9.,8.5));
#92215=CARTESIAN_POINT('',(90.5,8.5,9.));
#92216=CARTESIAN_POINT('',(90.,8.5,9.));
#92217=CARTESIAN_POINT('',(90.5,9.,8.5));
#92218=CARTESIAN_POINT('',(90.5,8.5,9.));
#92219=CARTESIAN_POINT('',(97.5786925113412,9.,8.5));
#92220=CARTESIAN_POINT('',(90.,9.,8.5));
#92221=CARTESIAN_POINT('',(98.4213074886588,9.,8.5));
#92222=CARTESIAN_POINT('Ctrl Pts',(98.4213074886588,9.,8.5));
#92223=CARTESIAN_POINT('Ctrl Pts',(98.,8.95,8.55));
#92224=CARTESIAN_POINT('Ctrl Pts',(97.5786925113412,9.,8.5));
#92225=CARTESIAN_POINT('',(108.431561285864,9.,8.5));
#92226=CARTESIAN_POINT('',(90.,9.,8.5));
#92227=CARTESIAN_POINT('Ctrl Pts',(110.,8.7,8.8));
#92228=CARTESIAN_POINT('Ctrl Pts',(109.215780642932,8.7,8.8));
#92229=CARTESIAN_POINT('Ctrl Pts',(108.431561285864,9.,8.5));
#92230=CARTESIAN_POINT('',(90.,9.,8.5));
#92231=CARTESIAN_POINT('Origin',(122.,10.75,8.5));
#92232=CARTESIAN_POINT('',(120.45,10.75,15.497705265805));
#92233=CARTESIAN_POINT('',(120.45,10.75,8.5));
#92234=CARTESIAN_POINT('Origin',(122.,10.75,15.497705265805));
#92235=CARTESIAN_POINT('Origin',(98.,10.75,8.625));
#92236=CARTESIAN_POINT('',(96.2,10.75,8.5));
#92237=CARTESIAN_POINT('Origin',(98.,10.75,8.5));
#92238=CARTESIAN_POINT('',(96.45,10.75,8.75));
#92239=CARTESIAN_POINT('',(96.325,10.75,8.625));
#92240=CARTESIAN_POINT('Origin',(98.,10.75,8.75));
#92241=CARTESIAN_POINT('Origin',(98.,10.75,8.5));
#92242=CARTESIAN_POINT('Origin',(98.,10.75,8.5));
#92243=CARTESIAN_POINT('',(96.45,10.75,15.497705265805));
#92244=CARTESIAN_POINT('',(96.45,10.75,8.5));
#92245=CARTESIAN_POINT('Origin',(98.,10.75,15.497705265805));
#92246=CARTESIAN_POINT('Origin',(110.,10.75,8.65));
#92247=CARTESIAN_POINT('Origin',(110.,10.75,8.8));
#92248=CARTESIAN_POINT('Origin',(110.,10.75,8.5));
#92249=CARTESIAN_POINT('Origin',(110.,10.75,8.5));
#92250=CARTESIAN_POINT('',(107.95,10.75,15.497705265805));
#92251=CARTESIAN_POINT('',(107.95,10.75,8.5));
#92252=CARTESIAN_POINT('Origin',(110.,10.75,15.497705265805));
#92253=CARTESIAN_POINT('Origin',(90.,8.5,8.5));
#92254=CARTESIAN_POINT('',(90.5,27.5,8.5));
#92255=CARTESIAN_POINT('',(90.5,13.375,8.5));
#92256=CARTESIAN_POINT('',(129.5,27.5,8.5));
#92257=CARTESIAN_POINT('',(90.,27.5,8.5));
#92258=CARTESIAN_POINT('',(129.5,13.375,8.5));
#92259=CARTESIAN_POINT('Origin',(110.,27.925,47.));
#92260=CARTESIAN_POINT('',(109.336675041929,28.,48.));
#92261=CARTESIAN_POINT('',(110.663324958071,28.,48.));
#92262=CARTESIAN_POINT('Ctrl Pts',(109.336675041929,28.,48.));
#92263=CARTESIAN_POINT('Ctrl Pts',(110.,27.8,48.2));
#92264=CARTESIAN_POINT('Ctrl Pts',(110.663324958071,28.,48.));
#92265=CARTESIAN_POINT('',(108.8,28.,47.));
#92266=CARTESIAN_POINT('Origin',(110.,28.,47.));
#92267=CARTESIAN_POINT('',(108.95,27.85,47.));
#92268=CARTESIAN_POINT('',(108.875,27.925,47.));
#92269=CARTESIAN_POINT('Origin',(110.,27.85,47.));
#92270=CARTESIAN_POINT('Origin',(110.,28.,47.));
#92271=CARTESIAN_POINT('Origin',(90.,27.75,48.25));
#92272=CARTESIAN_POINT('',(90.5,28.,48.));
#92273=CARTESIAN_POINT('',(90.,28.,48.));
#92274=CARTESIAN_POINT('',(90.5,28.,48.));
#92275=CARTESIAN_POINT('',(129.5,28.,48.));
#92276=CARTESIAN_POINT('',(129.5,27.5,48.5));
#92277=CARTESIAN_POINT('',(90.,28.,48.));
#92278=CARTESIAN_POINT('Origin',(110.,28.,47.));
#92279=CARTESIAN_POINT('',(108.95,22.8,47.));
#92280=CARTESIAN_POINT('',(108.95,28.,47.));
#92281=CARTESIAN_POINT('',(110.,22.8,45.95));
#92282=CARTESIAN_POINT('Origin',(110.,22.8,47.));
#92283=CARTESIAN_POINT('',(110.,22.8,48.05));
#92284=CARTESIAN_POINT('Origin',(110.,22.8,47.));
#92285=CARTESIAN_POINT('Origin',(110.,22.8,47.));
#92286=CARTESIAN_POINT('Origin',(110.,27.925,44.5));
#92287=CARTESIAN_POINT('',(108.8,28.,44.5));
#92288=CARTESIAN_POINT('Origin',(110.,28.,44.5));
#92289=CARTESIAN_POINT('',(108.95,27.85,44.5));
#92290=CARTESIAN_POINT('',(108.875,27.925,44.5));
#92291=CARTESIAN_POINT('Origin',(110.,27.85,44.5));
#92292=CARTESIAN_POINT('Origin',(90.,28.,8.5));
#92293=CARTESIAN_POINT('',(129.5,28.,9.));
#92294=CARTESIAN_POINT('',(129.5,28.,18.5));
#92295=CARTESIAN_POINT('',(90.5,28.,9.));
#92296=CARTESIAN_POINT('',(90.,28.,9.));
#92297=CARTESIAN_POINT('',(90.5,28.,18.5));
#92298=CARTESIAN_POINT('',(108.8,28.,42.));
#92299=CARTESIAN_POINT('Origin',(110.,28.,42.));
#92300=CARTESIAN_POINT('',(124.2,28.,44.5));
#92301=CARTESIAN_POINT('Origin',(126.,28.,44.5));
#92302=CARTESIAN_POINT('',(92.2,28.,44.5));
#92303=CARTESIAN_POINT('Origin',(94.,28.,44.5));
#92304=CARTESIAN_POINT('',(124.2,28.,12.5));
#92305=CARTESIAN_POINT('Origin',(126.,28.,12.5));
#92306=CARTESIAN_POINT('',(92.2,28.,12.5));
#92307=CARTESIAN_POINT('Origin',(94.,28.,12.5));
#92308=CARTESIAN_POINT('Origin',(110.,28.,44.5));
#92309=CARTESIAN_POINT('',(108.95,22.8,44.5));
#92310=CARTESIAN_POINT('',(108.95,28.,44.5));
#92311=CARTESIAN_POINT('',(110.,22.8,43.45));
#92312=CARTESIAN_POINT('Origin',(110.,22.8,44.5));
#92313=CARTESIAN_POINT('',(110.,22.8,45.55));
#92314=CARTESIAN_POINT('Origin',(110.,22.8,44.5));
#92315=CARTESIAN_POINT('Origin',(110.,22.8,44.5));
#92316=CARTESIAN_POINT('Origin',(110.,27.925,42.));
#92317=CARTESIAN_POINT('',(108.95,27.85,42.));
#92318=CARTESIAN_POINT('',(108.875,27.925,42.));
#92319=CARTESIAN_POINT('Origin',(110.,27.85,42.));
#92320=CARTESIAN_POINT('Origin',(110.,28.,42.));
#92321=CARTESIAN_POINT('',(108.95,22.8,42.));
#92322=CARTESIAN_POINT('',(108.95,28.,42.));
#92323=CARTESIAN_POINT('',(110.,22.8,40.95));
#92324=CARTESIAN_POINT('Origin',(110.,22.8,42.));
#92325=CARTESIAN_POINT('',(110.,22.8,43.05));
#92326=CARTESIAN_POINT('Origin',(110.,22.8,42.));
#92327=CARTESIAN_POINT('Origin',(110.,22.8,42.));
#92328=CARTESIAN_POINT('Origin',(110.,22.8,42.));
#92329=CARTESIAN_POINT('',(110.,22.8,48.5));
#92330=CARTESIAN_POINT('Origin',(110.,22.8,42.));
#92331=CARTESIAN_POINT('',(110.,22.8,48.5));
#92332=CARTESIAN_POINT('Origin',(110.,22.8,44.5));
#92333=CARTESIAN_POINT('',(110.,22.8,48.5));
#92334=CARTESIAN_POINT('Origin',(110.,22.8,44.5));
#92335=CARTESIAN_POINT('',(110.,22.8,48.5));
#92336=CARTESIAN_POINT('Origin',(110.,22.8,47.));
#92337=CARTESIAN_POINT('',(110.,22.8,48.5));
#92338=CARTESIAN_POINT('Origin',(110.,22.8,47.));
#92339=CARTESIAN_POINT('',(110.,22.8,48.5));
#92340=CARTESIAN_POINT('Origin',(126.,27.875,44.5));
#92341=CARTESIAN_POINT('',(124.45,27.75,44.5));
#92342=CARTESIAN_POINT('',(124.325,27.875,44.5));
#92343=CARTESIAN_POINT('Origin',(126.,27.75,44.5));
#92344=CARTESIAN_POINT('Origin',(126.,28.,44.5));
#92345=CARTESIAN_POINT('',(124.45,22.,44.5));
#92346=CARTESIAN_POINT('',(124.45,28.,44.5));
#92347=CARTESIAN_POINT('Origin',(126.,22.,44.5));
#92348=CARTESIAN_POINT('Origin',(94.,27.875,12.5));
#92349=CARTESIAN_POINT('',(92.45,27.75,12.5));
#92350=CARTESIAN_POINT('',(92.325,27.875,12.5));
#92351=CARTESIAN_POINT('Origin',(94.,27.75,12.5));
#92352=CARTESIAN_POINT('Origin',(94.,28.,12.5));
#92353=CARTESIAN_POINT('',(92.45,22.,12.5));
#92354=CARTESIAN_POINT('',(92.45,28.,12.5));
#92355=CARTESIAN_POINT('Origin',(94.,22.,12.5));
#92356=CARTESIAN_POINT('Origin',(94.,27.875,44.5));
#92357=CARTESIAN_POINT('',(92.45,27.75,44.5));
#92358=CARTESIAN_POINT('',(92.325,27.875,44.5));
#92359=CARTESIAN_POINT('Origin',(94.,27.75,44.5));
#92360=CARTESIAN_POINT('Origin',(94.,28.,44.5));
#92361=CARTESIAN_POINT('',(92.45,22.,44.5));
#92362=CARTESIAN_POINT('',(92.45,28.,44.5));
#92363=CARTESIAN_POINT('Origin',(94.,22.,44.5));
#92364=CARTESIAN_POINT('Origin',(126.,27.875,12.5));
#92365=CARTESIAN_POINT('',(124.45,27.75,12.5));
#92366=CARTESIAN_POINT('',(124.325,27.875,12.5));
#92367=CARTESIAN_POINT('Origin',(126.,27.75,12.5));
#92368=CARTESIAN_POINT('Origin',(126.,28.,12.5));
#92369=CARTESIAN_POINT('',(124.45,22.,12.5));
#92370=CARTESIAN_POINT('',(124.45,28.,12.5));
#92371=CARTESIAN_POINT('Origin',(126.,22.,12.5));
#92372=CARTESIAN_POINT('Origin',(126.,22.,44.5));
#92373=CARTESIAN_POINT('',(126.,21.0686660405073,44.5));
#92374=CARTESIAN_POINT('',(124.45,22.,44.5));
#92375=CARTESIAN_POINT('Origin',(126.,22.,12.5));
#92376=CARTESIAN_POINT('',(126.,21.0686660405073,12.5));
#92377=CARTESIAN_POINT('',(124.45,22.,12.5));
#92378=CARTESIAN_POINT('Origin',(94.,22.,44.5));
#92379=CARTESIAN_POINT('',(94.,21.0686660405073,44.5));
#92380=CARTESIAN_POINT('',(92.45,22.,44.5));
#92381=CARTESIAN_POINT('Origin',(94.,22.,12.5));
#92382=CARTESIAN_POINT('',(94.,21.0686660405073,12.5));
#92383=CARTESIAN_POINT('',(92.45,22.,12.5));
#92384=CARTESIAN_POINT('Origin',(110.,18.,48.35));
#92385=CARTESIAN_POINT('',(105.2,18.,48.2));
#92386=CARTESIAN_POINT('',(105.05,18.,48.35));
#92387=CARTESIAN_POINT('',(110.,22.8,48.2));
#92388=CARTESIAN_POINT('Origin',(110.,18.,48.2));
#92389=CARTESIAN_POINT('Origin',(110.,18.,48.2));
#92390=CARTESIAN_POINT('Origin',(110.,18.,48.5));
#92391=CARTESIAN_POINT('',(110.,22.8,48.5));
#92392=CARTESIAN_POINT('',(110.,22.8,48.5));
#92393=CARTESIAN_POINT('',(110.,22.8,48.5));
#92394=CARTESIAN_POINT('',(110.,22.8,25.8));
#92395=CARTESIAN_POINT('',(110.,22.8,48.5));
#92396=CARTESIAN_POINT('',(113.746998799039,15.,25.8));
#92397=CARTESIAN_POINT('Origin',(110.,18.,25.8));
#92398=CARTESIAN_POINT('',(113.746998799039,15.,32.));
#92399=CARTESIAN_POINT('',(113.746998799039,15.,48.5));
#92400=CARTESIAN_POINT('',(106.253001200961,15.,32.));
#92401=CARTESIAN_POINT('Origin',(110.,18.,32.));
#92402=CARTESIAN_POINT('',(106.253001200961,15.,25.8));
#92403=CARTESIAN_POINT('',(106.253001200961,15.,48.5));
#92404=CARTESIAN_POINT('Origin',(110.,18.,25.8));
#92405=CARTESIAN_POINT('Origin',(110.,18.,10.7414134684777));
#92406=CARTESIAN_POINT('',(110.,18.,9.98282693695541));
#92407=CARTESIAN_POINT('',(107.475,18.,11.5));
#92408=CARTESIAN_POINT('',(108.7375,18.,10.7414134684777));
#92409=CARTESIAN_POINT('Origin',(110.,18.,11.5));
#92410=CARTESIAN_POINT('Origin',(110.,18.,25.8));
#92411=CARTESIAN_POINT('',(107.475,18.,25.8));
#92412=CARTESIAN_POINT('Origin',(110.,18.,25.8));
#92413=CARTESIAN_POINT('',(107.475,18.,25.8));
#92414=CARTESIAN_POINT('Origin',(110.,18.,25.8));
#92415=CARTESIAN_POINT('',(100.,15.,25.8));
#92416=CARTESIAN_POINT('Origin',(90.,15.,25.));
#92417=CARTESIAN_POINT('',(90.,15.,32.));
#92418=CARTESIAN_POINT('',(90.,15.,32.));
#92419=CARTESIAN_POINT('',(90.,15.,25.));
#92420=CARTESIAN_POINT('',(90.,15.,26.75));
#92421=CARTESIAN_POINT('',(130.,15.,25.));
#92422=CARTESIAN_POINT('',(90.,15.,25.));
#92423=CARTESIAN_POINT('',(130.,15.,32.));
#92424=CARTESIAN_POINT('',(130.,15.,26.75));
#92425=CARTESIAN_POINT('',(90.,15.,32.));
#92426=CARTESIAN_POINT('Origin',(90.,7.5,25.));
#92427=CARTESIAN_POINT('',(130.,13.03,25.));
#92428=CARTESIAN_POINT('',(90.,13.03,25.));
#92429=CARTESIAN_POINT('',(90.,13.03,25.));
#92430=CARTESIAN_POINT('',(130.,12.875,25.));
#92431=CARTESIAN_POINT('',(90.,12.875,25.));
#92432=CARTESIAN_POINT('Origin',(90.,15.,32.));
#92433=CARTESIAN_POINT('',(130.,13.03,32.));
#92434=CARTESIAN_POINT('',(130.,16.625,32.));
#92435=CARTESIAN_POINT('',(90.,13.03,32.));
#92436=CARTESIAN_POINT('',(90.,13.03,32.));
#92437=CARTESIAN_POINT('',(90.,16.625,32.));
#92438=CARTESIAN_POINT('Origin',(90.,18.25,28.5));
#92439=CARTESIAN_POINT('',(90.,13.03,41.0519615242271));
#92440=CARTESIAN_POINT('',(90.,13.03,21.3406733260263));
#92441=CARTESIAN_POINT('',(90.,9.,38.7252399393929));
#92442=CARTESIAN_POINT('',(90.,12.2699206131736,40.6131294856374));
#92443=CARTESIAN_POINT('',(90.,9.,48.));
#92444=CARTESIAN_POINT('',(90.,9.,38.5));
#92445=CARTESIAN_POINT('',(90.,27.5,48.));
#92446=CARTESIAN_POINT('',(90.,23.125,48.));
#92447=CARTESIAN_POINT('',(90.,27.5,9.));
#92448=CARTESIAN_POINT('',(90.,27.5,18.5));
#92449=CARTESIAN_POINT('',(90.,9.,9.));
#92450=CARTESIAN_POINT('',(90.,13.375,9.));
#92451=CARTESIAN_POINT('',(90.,9.,16.5080682368869));
#92452=CARTESIAN_POINT('',(90.,9.,38.5));
#92453=CARTESIAN_POINT('',(90.,13.03,14.1813466520527));
#92454=CARTESIAN_POINT('',(90.,9.12242061317363,16.4373886629167));
#92455=CARTESIAN_POINT('',(90.,13.03,21.3406733260263));
#92456=CARTESIAN_POINT('Origin',(90.,13.03,14.1813466520527));
#92457=CARTESIAN_POINT('',(130.,13.03,41.0519615242271));
#92458=CARTESIAN_POINT('',(130.,13.03,21.3406733260263));
#92459=CARTESIAN_POINT('',(90.,13.03,41.0519615242271));
#92460=CARTESIAN_POINT('Origin',(90.,13.03,41.0519615242271));
#92461=CARTESIAN_POINT('',(90.5,8.5,38.4365648047981));
#92462=CARTESIAN_POINT('',(88.9835805013516,10.0164194986484,39.3120700105471));
#92463=CARTESIAN_POINT('',(130.,9.,38.7252399393929));
#92464=CARTESIAN_POINT('',(130.,12.2699206131736,40.6131294856374));
#92465=CARTESIAN_POINT('',(129.5,8.5,38.4365648047981));
#92466=CARTESIAN_POINT('',(122.44499092722,1.44499092721981,34.3633534174932));
#92467=CARTESIAN_POINT('',(90.,8.5,38.4365648047981));
#92468=CARTESIAN_POINT('Origin',(90.,7.5,17.3740936406713));
#92469=CARTESIAN_POINT('',(90.5,8.5,16.7967433714817));
#92470=CARTESIAN_POINT('',(93.25651022645,5.74348977355006,18.3882152927465));
#92471=CARTESIAN_POINT('',(129.5,8.5,16.7967433714817));
#92472=CARTESIAN_POINT('',(90.,8.5,16.7967433714817));
#92473=CARTESIAN_POINT('',(130.,9.,16.5080682368869));
#92474=CARTESIAN_POINT('',(118.172061202121,-2.82793879787853,23.3369318858005));
#92475=CARTESIAN_POINT('',(130.,13.03,14.1813466520527));
#92476=CARTESIAN_POINT('',(130.,9.12242061317363,16.4373886629167));
#92477=CARTESIAN_POINT('',(90.,13.03,14.1813466520527));
#92478=CARTESIAN_POINT('Origin',(90.,13.03,14.1813466520527));
#92479=CARTESIAN_POINT('',(130.,13.03,21.3406733260263));
#92480=CARTESIAN_POINT('Origin',(90.25,8.75,38.5));
#92481=CARTESIAN_POINT('',(90.5,8.5,48.));
#92482=CARTESIAN_POINT('',(90.5,8.5,38.5));
#92483=CARTESIAN_POINT('',(90.5,8.5,48.));
#92484=CARTESIAN_POINT('Origin',(90.25,8.75,38.5));
#92485=CARTESIAN_POINT('',(90.,9.,9.));
#92486=CARTESIAN_POINT('',(90.5,8.5,38.5));
#92487=CARTESIAN_POINT('Origin',(90.,8.5,48.5));
#92488=CARTESIAN_POINT('',(129.5,8.5,48.));
#92489=CARTESIAN_POINT('',(129.5,8.5,38.5));
#92490=CARTESIAN_POINT('',(90.,8.5,48.));
#92491=CARTESIAN_POINT('Origin',(129.75,8.75,38.5));
#92492=CARTESIAN_POINT('',(130.,9.,48.));
#92493=CARTESIAN_POINT('',(130.,9.,38.5));
#92494=CARTESIAN_POINT('',(130.,9.,48.));
#92495=CARTESIAN_POINT('Origin',(129.5,8.5,48.));
#92496=CARTESIAN_POINT('',(129.5,9.,48.5));
#92497=CARTESIAN_POINT('',(129.5,8.5,48.));
#92498=CARTESIAN_POINT('Origin',(129.5,27.5,48.5));
#92499=CARTESIAN_POINT('',(130.,27.5,48.));
#92500=CARTESIAN_POINT('',(129.5,28.,48.));
#92501=CARTESIAN_POINT('',(130.,27.5,48.));
#92502=CARTESIAN_POINT('Origin',(90.,9.,48.));
#92503=CARTESIAN_POINT('',(90.5,9.,48.5));
#92504=CARTESIAN_POINT('',(90.,9.,48.));
#92505=CARTESIAN_POINT('Origin',(129.5,9.,8.5));
#92506=CARTESIAN_POINT('',(130.,9.,9.));
#92507=CARTESIAN_POINT('',(129.5,8.5,9.));
#92508=CARTESIAN_POINT('',(130.,9.,9.));
#92509=CARTESIAN_POINT('Origin',(90.,27.5,48.));
#92510=CARTESIAN_POINT('',(90.,27.5,48.));
#92511=CARTESIAN_POINT('',(90.5,27.5,48.5));
#92512=CARTESIAN_POINT('Origin',(129.5,28.,9.));
#92513=CARTESIAN_POINT('',(130.,27.5,9.));
#92514=CARTESIAN_POINT('',(129.5,27.5,8.5));
#92515=CARTESIAN_POINT('',(129.5,28.,9.));
#92516=CARTESIAN_POINT('',(130.,27.5,9.));
#92517=CARTESIAN_POINT('Origin',(90.,9.,9.));
#92518=CARTESIAN_POINT('',(90.5,9.,8.5));
#92519=CARTESIAN_POINT('Origin',(90.5,28.,9.));
#92520=CARTESIAN_POINT('',(90.,27.5,9.));
#92521=CARTESIAN_POINT('',(90.5,28.,9.));
#92522=CARTESIAN_POINT('',(90.5,27.5,8.5));
#92523=CARTESIAN_POINT('Origin',(90.25,27.75,18.5));
#92524=CARTESIAN_POINT('Origin',(90.,27.75,8.75));
#92525=CARTESIAN_POINT('Origin',(90.25,13.375,8.75));
#92526=CARTESIAN_POINT('Origin',(129.75,27.75,18.5));
#92527=CARTESIAN_POINT('',(130.,27.5,18.5));
#92528=CARTESIAN_POINT('Origin',(129.75,13.375,8.75));
#92529=CARTESIAN_POINT('',(130.,13.375,9.));
#92530=CARTESIAN_POINT('Origin',(90.25,23.125,48.25));
#92531=CARTESIAN_POINT('Origin',(129.75,8.75,38.5));
#92532=CARTESIAN_POINT('',(129.5,8.5,38.5));
#92533=CARTESIAN_POINT('',(130.,9.,38.5));
#92534=CARTESIAN_POINT('Origin',(90.,8.75,48.25));
#92535=CARTESIAN_POINT('Origin',(129.75,23.125,48.25));
#92536=CARTESIAN_POINT('',(130.,23.125,48.));
#92537=CARTESIAN_POINT('Origin',(90.,8.5,48.5));
#92538=CARTESIAN_POINT('Origin',(130.,18.25,28.5));
#113947=UNCERTAINTY_MEASURE_WITH_UNIT(LENGTH_MEASURE(0.01),#113985,
'DISTANCE_ACCURACY_VALUE',
'Maximum model space distance between geometric entities at asserted c
onnectivities');
#113964=UNCERTAINTY_MEASURE_WITH_UNIT(LENGTH_MEASURE(0.01),#113985,
'DISTANCE_ACCURACY_VALUE',
'Maximum model space distance between geometric entities at asserted c
onnectivities');
#113967=(
GEOMETRIC_REPRESENTATION_CONTEXT(3)
GLOBAL_UNCERTAINTY_ASSIGNED_CONTEXT((#113947))
GLOBAL_UNIT_ASSIGNED_CONTEXT((#113985,#113987,#113988))
REPRESENTATION_CONTEXT('','3D')
);
#113984=(
GEOMETRIC_REPRESENTATION_CONTEXT(3)
GLOBAL_UNCERTAINTY_ASSIGNED_CONTEXT((#113964))
GLOBAL_UNIT_ASSIGNED_CONTEXT((#113985,#113987,#113988))
REPRESENTATION_CONTEXT('','3D')
);
#113985=(
LENGTH_UNIT()
NAMED_UNIT(*)
SI_UNIT(.MILLI.,.METRE.)
);
#113987=(
NAMED_UNIT(*)
PLANE_ANGLE_UNIT()
SI_UNIT($,.RADIAN.)
);
#113988=(
NAMED_UNIT(*)
SI_UNIT($,.STERADIAN.)
SOLID_ANGLE_UNIT()
);
#113991=SHAPE_DEFINITION_REPRESENTATION(#114010,#114053);
#114010=PRODUCT_DEFINITION_SHAPE('',$,#114073);
#114053=SHAPE_REPRESENTATION('',(#61812),#113967);
#114070=PRODUCT_DEFINITION_CONTEXT('part definition',#114129,'design');
#114073=PRODUCT_DEFINITION('2026-10-05-09-48-36-190',
'Machined Alloy Sliding Carriage 40 x 40',#114092,#114070);
#114092=PRODUCT_DEFINITION_FORMATION('',$,#114133);
#114129=APPLICATION_CONTEXT(
'Core Data for Automotive Mechanical Design Process');
#114130=PRODUCT_CONTEXT('part definition',#114129,'mechanical');
#114133=PRODUCT('2026-10-05-09-48-36-190',
'Machined Alloy Sliding Carriage 40 x 40',$,(#114130));
#114318=COLOUR_RGB('Off White',0.89,0.88,0.83);
#114319=FILL_AREA_STYLE_COLOUR('',#114318);
#114320=FILL_AREA_STYLE('',(#114319));
#114321=SURFACE_STYLE_FILL_AREA(#114320);
#114322=SURFACE_SIDE_STYLE('',(#114321));
#114323=SURFACE_STYLE_USAGE(.BOTH.,#114322);
#114324=PRESENTATION_STYLE_ASSIGNMENT((#114323));
ENDSEC;
END-ISO-10303-21;
